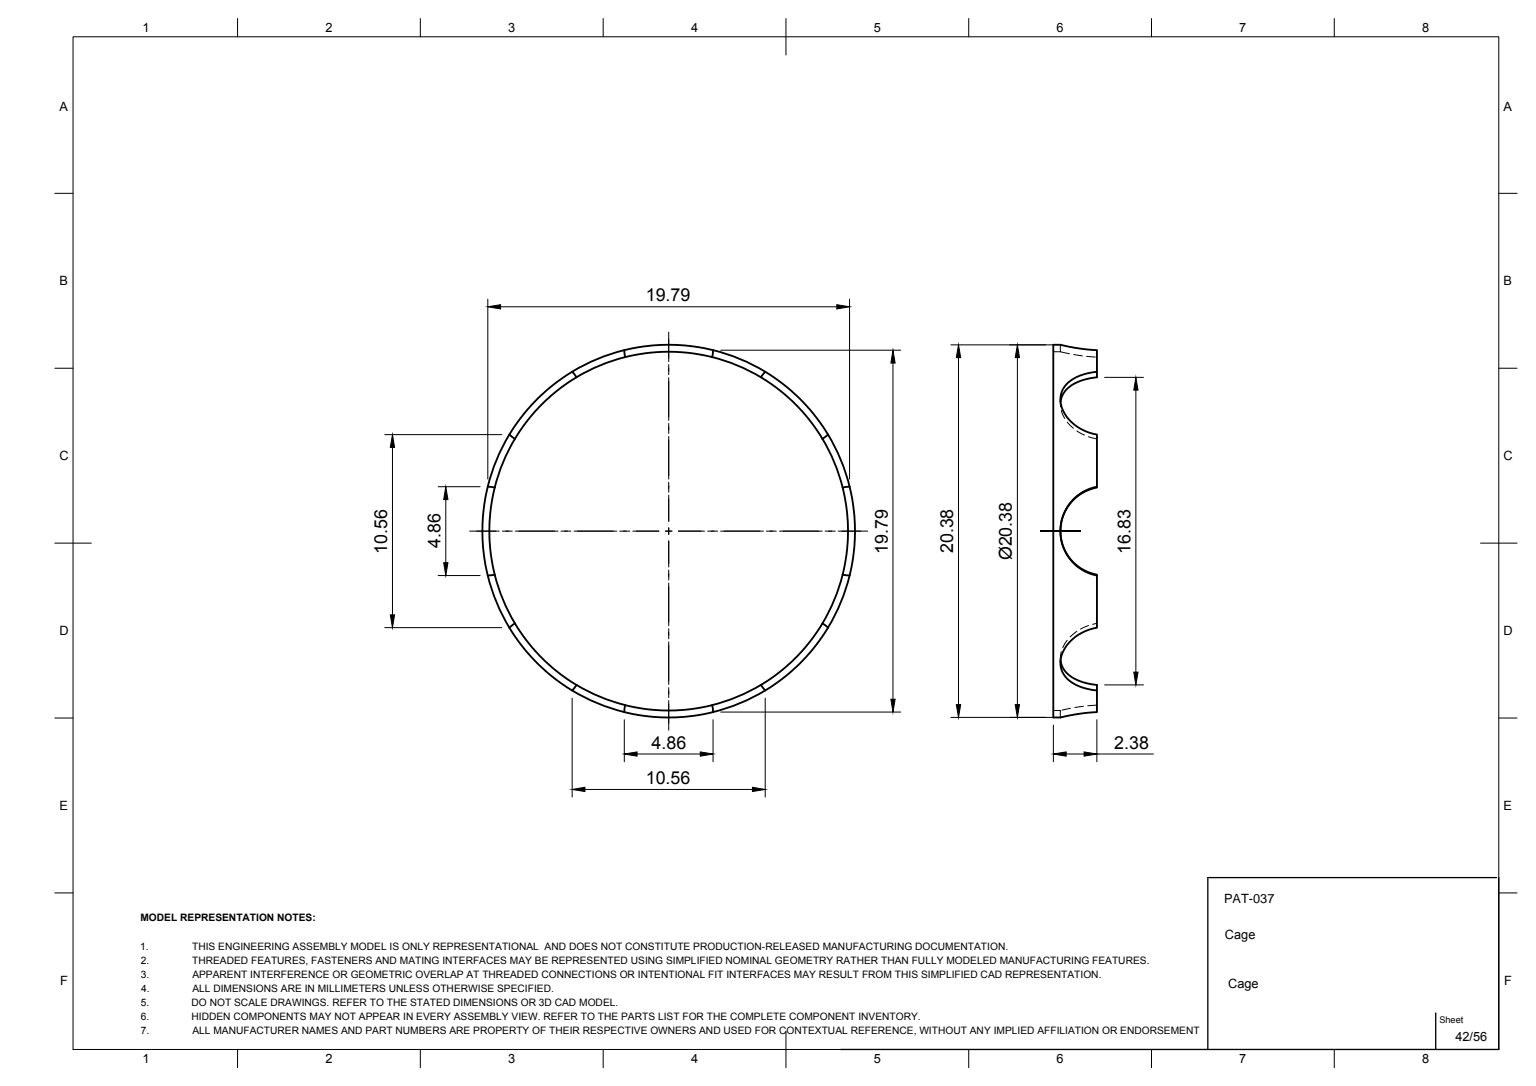
ISO-10303-21;
HEADER;
/* Generated by software containing ST-Developer
 * from STEP Tools, Inc. (www.steptools.com) 
 */

FILE_DESCRIPTION(
/* description */ ('Flywheel Crank-Slider'),
/* implementation_level */ '2;1');

FILE_NAME(
/* name */ 'Cage.step',
/* time_stamp */ '2026-10-28T03:23:13-07:00',
/* author */ (''),
/* organization */ (''),
/* preprocessor_version */ 'ST-DEVELOPER v20.2',
/* originating_system */ 'Autodesk Translation Framework v15.17.0.0',
/* authorisation */ '');

FILE_SCHEMA (('AUTOMOTIVE_DESIGN { 1 0 10303 214 3 1 1 }'));
ENDSEC;

DATA;
#10=MECHANICAL_DESIGN_GEOMETRIC_PRESENTATION_REPRESENTATION('',(#716),#17322);
#493=B_SPLINE_CURVE_WITH_KNOTS('',3,(#16156,#16157,#16158,#16159,#16160,
#16161,#16162,#16163,#16164,#16165,#16166,#16167,#16168,#16169,#16170,#16171,
#16172,#16173,#16174,#16175,#16176,#16177),.UNSPECIFIED.,.F.,.F.,(4,2,2,
2,2,2,2,2,2,2,4),(0.0473477652366656,0.126350602536658,0.189525903804987,
0.252701205073317,0.313298422430275,0.373895639787233,0.434492857144191,
0.495090074501149,0.558265375769478,0.621440677037807,0.7004435143378),
 .UNSPECIFIED.);
#494=B_SPLINE_CURVE_WITH_KNOTS('',3,(#16181,#16182,#16183,#16184,#16185,
#16186,#16187,#16188,#16189,#16190,#16191,#16192,#16193,#16194,#16195,#16196,
#16197,#16198,#16199,#16200,#16201,#16202),.UNSPECIFIED.,.F.,.F.,(4,2,2,
2,2,2,2,2,2,2,4),(0.0464897534940957,0.0852567806515119,0.170513561303024,
0.246687263103517,0.308657850341199,0.370628437578881,0.432599024816563,
0.494569612054245,0.570743313854739,0.656000094506251,0.694767121663666),
 .UNSPECIFIED.);
#495=B_SPLINE_CURVE_WITH_KNOTS('',3,(#16208,#16209,#16210,#16211,#16212,
#16213,#16214,#16215,#16216,#16217,#16218,#16219,#16220,#16221,#16222,#16223,
#16224,#16225,#16226,#16227,#16228,#16229),.UNSPECIFIED.,.F.,.F.,(4,2,2,
2,2,2,2,2,2,2,4),(0.0464897534940957,0.0852567806515118,0.170513561303024,
0.246687263103517,0.308657850341199,0.370628437578881,0.432599024816563,
0.494569612054245,0.570743313854738,0.65600009450625,0.694767121663666),
 .UNSPECIFIED.);
#496=B_SPLINE_CURVE_WITH_KNOTS('',3,(#16233,#16234,#16235,#16236,#16237,
#16238,#16239,#16240,#16241,#16242,#16243,#16244,#16245,#16246,#16247,#16248,
#16249,#16250,#16251,#16252,#16253,#16254),.UNSPECIFIED.,.F.,.F.,(4,2,2,
2,2,2,2,2,2,2,4),(0.0464897534940957,0.0852567806515119,0.170513561303024,
0.246687263103517,0.308657850341199,0.370628437578881,0.432599024816563,
0.494569612054245,0.570743313854739,0.656000094506251,0.694767121663666),
 .UNSPECIFIED.);
#497=B_SPLINE_CURVE_WITH_KNOTS('',3,(#16258,#16259,#16260,#16261,#16262,
#16263,#16264,#16265,#16266,#16267,#16268,#16269),.UNSPECIFIED.,.F.,.F.,
(4,2,2,2,2,4),(0.0464897534940957,0.0852567806515119,0.170513561303024,
0.246687263103517,0.308657850341199,0.370628437578881),.UNSPECIFIED.);
#498=B_SPLINE_CURVE_WITH_KNOTS('',3,(#16274,#16275,#16276,#16277,#16278,
#16279,#16280,#16281,#16282,#16283,#16284,#16285),.UNSPECIFIED.,.F.,.F.,
(4,2,2,2,2,4),(0.370628437578881,0.432599024816563,0.494569612054245,0.570743313854738,
0.65600009450625,0.694767121663666),.UNSPECIFIED.);
#499=B_SPLINE_CURVE_WITH_KNOTS('',3,(#16289,#16290,#16291,#16292,#16293,
#16294,#16295,#16296,#16297,#16298,#16299,#16300,#16301,#16302,#16303,#16304,
#16305,#16306,#16307,#16308,#16309,#16310),.UNSPECIFIED.,.F.,.F.,(4,2,2,
2,2,2,2,2,2,2,4),(0.0464897534940957,0.0852567806515121,0.170513561303024,
0.246687263103518,0.308657850341199,0.370628437578881,0.432599024816563,
0.494569612054245,0.570743313854738,0.65600009450625,0.694767121663666),
 .UNSPECIFIED.);
#500=B_SPLINE_CURVE_WITH_KNOTS('',3,(#16314,#16315,#16316,#16317,#16318,
#16319,#16320,#16321,#16322,#16323,#16324,#16325,#16326,#16327,#16328,#16329,
#16330,#16331,#16332,#16333,#16334,#16335),.UNSPECIFIED.,.F.,.F.,(4,2,2,
2,2,2,2,2,2,2,4),(0.0464897534940957,0.0852567806515119,0.170513561303024,
0.246687263103517,0.308657850341199,0.370628437578881,0.432599024816563,
0.494569612054245,0.570743313854738,0.65600009450625,0.694767121663667),
 .UNSPECIFIED.);
#501=B_SPLINE_CURVE_WITH_KNOTS('',3,(#16339,#16340,#16341,#16342,#16343,
#16344,#16345,#16346,#16347,#16348,#16349,#16350,#16351,#16352,#16353,#16354,
#16355,#16356,#16357,#16358,#16359,#16360),.UNSPECIFIED.,.F.,.F.,(4,2,2,
2,2,2,2,2,2,2,4),(0.0464897534940957,0.0852567806515119,0.170513561303024,
0.246687263103517,0.308657850341199,0.370628437578881,0.432599024816563,
0.494569612054245,0.570743313854738,0.65600009450625,0.694767121663666),
 .UNSPECIFIED.);
#502=B_SPLINE_CURVE_WITH_KNOTS('',3,(#16364,#16365,#16366,#16367,#16368,
#16369,#16370,#16371,#16372,#16373,#16374,#16375,#16376,#16377,#16378,#16379,
#16380,#16381,#16382,#16383,#16384,#16385),.UNSPECIFIED.,.F.,.F.,(4,2,2,
2,2,2,2,2,2,2,4),(0.0464897534940957,0.0852567806515119,0.170513561303024,
0.246687263103517,0.308657850341199,0.370628437578881,0.432599024816563,
0.494569612054245,0.570743313854739,0.656000094506251,0.694767121663667),
 .UNSPECIFIED.);
#503=B_SPLINE_CURVE_WITH_KNOTS('',3,(#16393,#16394,#16395,#16396,#16397,
#16398,#16399,#16400,#16401,#16402,#16403,#16404,#16405,#16406,#16407,#16408,
#16409,#16410,#16411,#16412,#16413,#16414),.UNSPECIFIED.,.F.,.F.,(4,2,2,
2,2,2,2,2,2,2,4),(0.0473477652366656,0.126350602536658,0.189525903804987,
0.252701205073316,0.313298422430274,0.373895639787232,0.434492857144191,
0.495090074501149,0.558265375769478,0.621440677037807,0.7004435143378),
 .UNSPECIFIED.);
#504=B_SPLINE_CURVE_WITH_KNOTS('',3,(#16422,#16423,#16424,#16425,#16426,
#16427,#16428,#16429,#16430,#16431,#16432,#16433,#16434,#16435,#16436,#16437,
#16438,#16439,#16440,#16441,#16442,#16443),.UNSPECIFIED.,.F.,.F.,(4,2,2,
2,2,2,2,2,2,2,4),(0.0473477652366656,0.126350602536658,0.189525903804987,
0.252701205073317,0.313298422430275,0.373895639787233,0.434492857144191,
0.495090074501149,0.558265375769478,0.621440677037807,0.7004435143378),
 .UNSPECIFIED.);
#505=B_SPLINE_CURVE_WITH_KNOTS('',3,(#16452,#16453,#16454,#16455,#16456,
#16457,#16458,#16459,#16460,#16461,#16462,#16463),.UNSPECIFIED.,.F.,.F.,
(4,2,2,2,2,4),(0.0473477652366656,0.126350602536658,0.189525903804987,0.252701205073316,
0.313298422430275,0.373895639787233),.UNSPECIFIED.);
#506=B_SPLINE_CURVE_WITH_KNOTS('',3,(#16465,#16466,#16467,#16468,#16469,
#16470,#16471,#16472,#16473,#16474,#16475,#16476),.UNSPECIFIED.,.F.,.F.,
(4,2,2,2,2,4),(0.373895639787233,0.434492857144191,0.495090074501149,0.558265375769478,
0.621440677037807,0.7004435143378),.UNSPECIFIED.);
#507=B_SPLINE_CURVE_WITH_KNOTS('',3,(#16483,#16484,#16485,#16486,#16487,
#16488,#16489,#16490,#16491,#16492,#16493,#16494,#16495,#16496,#16497,#16498,
#16499,#16500,#16501,#16502,#16503,#16504),.UNSPECIFIED.,.F.,.F.,(4,2,2,
2,2,2,2,2,2,2,4),(0.0473477652366656,0.126350602536658,0.189525903804987,
0.252701205073316,0.313298422430275,0.373895639787233,0.434492857144191,
0.495090074501149,0.558265375769478,0.621440677037807,0.7004435143378),
 .UNSPECIFIED.);
#508=B_SPLINE_CURVE_WITH_KNOTS('',3,(#16512,#16513,#16514,#16515,#16516,
#16517,#16518,#16519,#16520,#16521,#16522,#16523,#16524,#16525,#16526,#16527,
#16528,#16529,#16530,#16531,#16532,#16533),.UNSPECIFIED.,.F.,.F.,(4,2,2,
2,2,2,2,2,2,2,4),(0.0473477652366656,0.126350602536658,0.189525903804987,
0.252701205073317,0.313298422430275,0.373895639787233,0.434492857144191,
0.495090074501149,0.558265375769478,0.621440677037807,0.7004435143378),
 .UNSPECIFIED.);
#509=B_SPLINE_CURVE_WITH_KNOTS('',3,(#16541,#16542,#16543,#16544,#16545,
#16546,#16547,#16548,#16549,#16550,#16551,#16552,#16553,#16554,#16555,#16556,
#16557,#16558,#16559,#16560,#16561,#16562),.UNSPECIFIED.,.F.,.F.,(4,2,2,
2,2,2,2,2,2,2,4),(0.0473477652366656,0.126350602536658,0.189525903804987,
0.252701205073316,0.313298422430275,0.373895639787233,0.434492857144191,
0.495090074501149,0.558265375769478,0.621440677037807,0.7004435143378),
 .UNSPECIFIED.);
#510=B_SPLINE_CURVE_WITH_KNOTS('',3,(#16571,#16572,#16573,#16574,#16575,
#16576,#16577,#16578,#16579,#16580,#16581,#16582,#16583,#16584,#16585,#16586,
#16587,#16588,#16589,#16590,#16591,#16592),.UNSPECIFIED.,.F.,.F.,(4,2,2,
2,2,2,2,2,2,2,4),(0.0473477652366656,0.126350602536658,0.189525903804987,
0.252701205073317,0.313298422430275,0.373895639787233,0.434492857144191,
0.495090074501149,0.558265375769478,0.621440677037807,0.7004435143378),
 .UNSPECIFIED.);
#521=SPHERICAL_SURFACE('',#10452,0.247676);
#522=SPHERICAL_SURFACE('',#10468,0.247676);
#523=SPHERICAL_SURFACE('',#10473,0.247676);
#524=SPHERICAL_SURFACE('',#10478,0.247676);
#525=SPHERICAL_SURFACE('',#10483,0.247676);
#526=SPHERICAL_SURFACE('',#10488,0.247676);
#527=SPHERICAL_SURFACE('',#10493,0.247676);
#528=SPHERICAL_SURFACE('',#10501,0.247676);
#604=SHAPE_REPRESENTATION_RELATIONSHIP('SRR','None',#17604,#656);
#656=ADVANCED_BREP_SHAPE_REPRESENTATION('',(#773),#17308);
#716=STYLED_ITEM('',(#17931),#773);
#773=MANIFOLD_SOLID_BREP('Continuous crown cage',#9098);
#947=FACE_BOUND('',#2441,.T.);
#1246=PLANE('',#10465);
#1247=PLANE('',#10470);
#1248=PLANE('',#10475);
#1249=PLANE('',#10480);
#1250=PLANE('',#10485);
#1251=PLANE('',#10490);
#1252=PLANE('',#10499);
#1253=PLANE('',#10503);
#1254=PLANE('',#10504);
#1726=FACE_OUTER_BOUND('',#2423,.T.);
#1727=FACE_OUTER_BOUND('',#2424,.T.);
#1728=FACE_OUTER_BOUND('',#2425,.T.);
#1729=FACE_OUTER_BOUND('',#2426,.T.);
#1730=FACE_OUTER_BOUND('',#2427,.T.);
#1731=FACE_OUTER_BOUND('',#2428,.T.);
#1732=FACE_OUTER_BOUND('',#2429,.T.);
#1733=FACE_OUTER_BOUND('',#2430,.T.);
#1734=FACE_OUTER_BOUND('',#2431,.T.);
#1735=FACE_OUTER_BOUND('',#2432,.T.);
#1736=FACE_OUTER_BOUND('',#2433,.T.);
#1737=FACE_OUTER_BOUND('',#2434,.T.);
#1738=FACE_OUTER_BOUND('',#2435,.T.);
#1739=FACE_OUTER_BOUND('',#2436,.T.);
#1740=FACE_OUTER_BOUND('',#2437,.T.);
#1741=FACE_OUTER_BOUND('',#2438,.T.);
#1742=FACE_OUTER_BOUND('',#2439,.T.);
#1743=FACE_OUTER_BOUND('',#2440,.T.);
#1744=FACE_OUTER_BOUND('',#2442,.T.);
#2423=EDGE_LOOP('',(#7778,#7779,#7780,#7781));
#2424=EDGE_LOOP('',(#7782,#7783,#7784,#7785,#7786,#7787,#7788,#7789,#7790,
#7791,#7792,#7793,#7794,#7795,#7796,#7797,#7798,#7799,#7800,#7801));
#2425=EDGE_LOOP('',(#7802,#7803,#7804,#7805));
#2426=EDGE_LOOP('',(#7806,#7807,#7808,#7809));
#2427=EDGE_LOOP('',(#7810,#7811,#7812,#7813));
#2428=EDGE_LOOP('',(#7814,#7815,#7816,#7817));
#2429=EDGE_LOOP('',(#7818,#7819,#7820,#7821));
#2430=EDGE_LOOP('',(#7822,#7823,#7824,#7825,#7826,#7827));
#2431=EDGE_LOOP('',(#7828,#7829,#7830,#7831));
#2432=EDGE_LOOP('',(#7832,#7833,#7834,#7835));
#2433=EDGE_LOOP('',(#7836,#7837,#7838,#7839));
#2434=EDGE_LOOP('',(#7840,#7841,#7842,#7843));
#2435=EDGE_LOOP('',(#7844,#7845,#7846,#7847));
#2436=EDGE_LOOP('',(#7848,#7849,#7850,#7851));
#2437=EDGE_LOOP('',(#7852,#7853,#7854,#7855,#7856,#7857,#7858,#7859,#7860,
#7861,#7862,#7863,#7864,#7865,#7866,#7867,#7868,#7869,#7870,#7871));
#2438=EDGE_LOOP('',(#7872,#7873,#7874,#7875));
#2439=EDGE_LOOP('',(#7876,#7877,#7878,#7879));
#2440=EDGE_LOOP('',(#7880));
#2441=EDGE_LOOP('',(#7881));
#2442=EDGE_LOOP('',(#7882,#7883,#7884,#7885));
#3096=LINE('',#16271,#3707);
#3097=LINE('',#16567,#3708);
#3707=VECTOR('',#12858,1.019052);
#3708=VECTOR('',#12935,0.980948);
#4150=CIRCLE('',#10453,0.243053047864041);
#4151=CIRCLE('',#10454,0.243053047864041);
#4152=CIRCLE('',#10456,1.019052);
#4153=CIRCLE('',#10457,1.019052);
#4154=CIRCLE('',#10458,1.019052);
#4155=CIRCLE('',#10459,1.019052);
#4156=CIRCLE('',#10460,1.019052);
#4157=CIRCLE('',#10461,1.019052);
#4158=CIRCLE('',#10462,1.019052);
#4159=CIRCLE('',#10463,1.019052);
#4160=CIRCLE('',#10464,1.019052);
#4161=CIRCLE('',#10466,0.980948);
#4162=CIRCLE('',#10467,0.243053047864041);
#4163=CIRCLE('',#10469,0.243053047864041);
#4164=CIRCLE('',#10471,0.980948);
#4165=CIRCLE('',#10472,0.243053047864041);
#4166=CIRCLE('',#10474,0.243053047864041);
#4167=CIRCLE('',#10476,0.980948);
#4168=CIRCLE('',#10477,0.243053047864041);
#4169=CIRCLE('',#10479,0.243053047864041);
#4170=CIRCLE('',#10481,0.980948);
#4171=CIRCLE('',#10482,0.243053047864041);
#4172=CIRCLE('',#10484,0.243053047864041);
#4173=CIRCLE('',#10486,0.980948);
#4174=CIRCLE('',#10487,0.243053047864041);
#4175=CIRCLE('',#10489,0.243053047864041);
#4176=CIRCLE('',#10491,0.980948);
#4177=CIRCLE('',#10492,0.243053047864041);
#4178=CIRCLE('',#10494,0.243053047864041);
#4179=CIRCLE('',#10496,0.980948);
#4180=CIRCLE('',#10497,0.980948);
#4181=CIRCLE('',#10498,0.980948);
#4182=CIRCLE('',#10500,0.243053047864041);
#4183=CIRCLE('',#10502,0.243053047864041);
#4835=VERTEX_POINT('',#16154);
#4836=VERTEX_POINT('',#16155);
#4837=VERTEX_POINT('',#16178);
#4838=VERTEX_POINT('',#16180);
#4839=VERTEX_POINT('',#16205);
#4840=VERTEX_POINT('',#16207);
#4841=VERTEX_POINT('',#16230);
#4842=VERTEX_POINT('',#16232);
#4843=VERTEX_POINT('',#16255);
#4844=VERTEX_POINT('',#16257);
#4845=VERTEX_POINT('',#16270);
#4846=VERTEX_POINT('',#16273);
#4847=VERTEX_POINT('',#16286);
#4848=VERTEX_POINT('',#16288);
#4849=VERTEX_POINT('',#16311);
#4850=VERTEX_POINT('',#16313);
#4851=VERTEX_POINT('',#16336);
#4852=VERTEX_POINT('',#16338);
#4853=VERTEX_POINT('',#16361);
#4854=VERTEX_POINT('',#16363);
#4855=VERTEX_POINT('',#16388);
#4856=VERTEX_POINT('',#16392);
#4857=VERTEX_POINT('',#16417);
#4858=VERTEX_POINT('',#16421);
#4859=VERTEX_POINT('',#16446);
#4860=VERTEX_POINT('',#16450);
#4861=VERTEX_POINT('',#16451);
#4862=VERTEX_POINT('',#16478);
#4863=VERTEX_POINT('',#16482);
#4864=VERTEX_POINT('',#16507);
#4865=VERTEX_POINT('',#16511);
#4866=VERTEX_POINT('',#16536);
#4867=VERTEX_POINT('',#16540);
#4868=VERTEX_POINT('',#16565);
#4869=VERTEX_POINT('',#16568);
#4870=VERTEX_POINT('',#16570);
#5846=EDGE_CURVE('',#4835,#4836,#493,.T.);
#5847=EDGE_CURVE('',#4837,#4835,#4150,.T.);
#5848=EDGE_CURVE('',#4838,#4837,#494,.T.);
#5849=EDGE_CURVE('',#4836,#4838,#4151,.T.);
#5850=EDGE_CURVE('',#4839,#4837,#4152,.T.);
#5851=EDGE_CURVE('',#4839,#4840,#495,.T.);
#5852=EDGE_CURVE('',#4841,#4840,#4153,.T.);
#5853=EDGE_CURVE('',#4841,#4842,#496,.T.);
#5854=EDGE_CURVE('',#4843,#4842,#4154,.T.);
#5855=EDGE_CURVE('',#4843,#4844,#497,.T.);
#5856=EDGE_CURVE('',#4844,#4845,#3096,.T.);
#5857=EDGE_CURVE('',#4845,#4845,#4155,.T.);
#5858=EDGE_CURVE('',#4844,#4846,#498,.T.);
#5859=EDGE_CURVE('',#4847,#4846,#4156,.T.);
#5860=EDGE_CURVE('',#4847,#4848,#499,.T.);
#5861=EDGE_CURVE('',#4849,#4848,#4157,.T.);
#5862=EDGE_CURVE('',#4849,#4850,#500,.T.);
#5863=EDGE_CURVE('',#4851,#4850,#4158,.T.);
#5864=EDGE_CURVE('',#4851,#4852,#501,.T.);
#5865=EDGE_CURVE('',#4853,#4852,#4159,.T.);
#5866=EDGE_CURVE('',#4853,#4854,#502,.T.);
#5867=EDGE_CURVE('',#4838,#4854,#4160,.T.);
#5868=EDGE_CURVE('',#4835,#4855,#4161,.T.);
#5869=EDGE_CURVE('',#4855,#4839,#4162,.T.);
#5870=EDGE_CURVE('',#4856,#4855,#503,.T.);
#5871=EDGE_CURVE('',#4840,#4856,#4163,.T.);
#5872=EDGE_CURVE('',#4856,#4857,#4164,.T.);
#5873=EDGE_CURVE('',#4857,#4841,#4165,.T.);
#5874=EDGE_CURVE('',#4858,#4857,#504,.T.);
#5875=EDGE_CURVE('',#4842,#4858,#4166,.T.);
#5876=EDGE_CURVE('',#4858,#4859,#4167,.T.);
#5877=EDGE_CURVE('',#4859,#4843,#4168,.T.);
#5878=EDGE_CURVE('',#4860,#4861,#505,.T.);
#5879=EDGE_CURVE('',#4846,#4860,#4169,.T.);
#5880=EDGE_CURVE('',#4861,#4859,#506,.T.);
#5881=EDGE_CURVE('',#4860,#4862,#4170,.T.);
#5882=EDGE_CURVE('',#4862,#4847,#4171,.T.);
#5883=EDGE_CURVE('',#4863,#4862,#507,.T.);
#5884=EDGE_CURVE('',#4848,#4863,#4172,.T.);
#5885=EDGE_CURVE('',#4863,#4864,#4173,.T.);
#5886=EDGE_CURVE('',#4864,#4849,#4174,.T.);
#5887=EDGE_CURVE('',#4865,#4864,#508,.T.);
#5888=EDGE_CURVE('',#4850,#4865,#4175,.T.);
#5889=EDGE_CURVE('',#4865,#4866,#4176,.T.);
#5890=EDGE_CURVE('',#4866,#4851,#4177,.T.);
#5891=EDGE_CURVE('',#4867,#4866,#509,.T.);
#5892=EDGE_CURVE('',#4852,#4867,#4178,.T.);
#5893=EDGE_CURVE('',#4868,#4868,#4179,.T.);
#5894=EDGE_CURVE('',#4868,#4861,#3097,.T.);
#5895=EDGE_CURVE('',#4869,#4836,#4180,.T.);
#5896=EDGE_CURVE('',#4869,#4870,#510,.T.);
#5897=EDGE_CURVE('',#4867,#4870,#4181,.T.);
#5898=EDGE_CURVE('',#4854,#4869,#4182,.T.);
#5899=EDGE_CURVE('',#4870,#4853,#4183,.T.);
#7778=ORIENTED_EDGE('',*,*,#5846,.F.);
#7779=ORIENTED_EDGE('',*,*,#5847,.F.);
#7780=ORIENTED_EDGE('',*,*,#5848,.F.);
#7781=ORIENTED_EDGE('',*,*,#5849,.F.);
#7782=ORIENTED_EDGE('',*,*,#5848,.T.);
#7783=ORIENTED_EDGE('',*,*,#5850,.F.);
#7784=ORIENTED_EDGE('',*,*,#5851,.T.);
#7785=ORIENTED_EDGE('',*,*,#5852,.F.);
#7786=ORIENTED_EDGE('',*,*,#5853,.T.);
#7787=ORIENTED_EDGE('',*,*,#5854,.F.);
#7788=ORIENTED_EDGE('',*,*,#5855,.T.);
#7789=ORIENTED_EDGE('',*,*,#5856,.T.);
#7790=ORIENTED_EDGE('',*,*,#5857,.F.);
#7791=ORIENTED_EDGE('',*,*,#5856,.F.);
#7792=ORIENTED_EDGE('',*,*,#5858,.T.);
#7793=ORIENTED_EDGE('',*,*,#5859,.F.);
#7794=ORIENTED_EDGE('',*,*,#5860,.T.);
#7795=ORIENTED_EDGE('',*,*,#5861,.F.);
#7796=ORIENTED_EDGE('',*,*,#5862,.T.);
#7797=ORIENTED_EDGE('',*,*,#5863,.F.);
#7798=ORIENTED_EDGE('',*,*,#5864,.T.);
#7799=ORIENTED_EDGE('',*,*,#5865,.F.);
#7800=ORIENTED_EDGE('',*,*,#5866,.T.);
#7801=ORIENTED_EDGE('',*,*,#5867,.F.);
#7802=ORIENTED_EDGE('',*,*,#5847,.T.);
#7803=ORIENTED_EDGE('',*,*,#5868,.T.);
#7804=ORIENTED_EDGE('',*,*,#5869,.T.);
#7805=ORIENTED_EDGE('',*,*,#5850,.T.);
#7806=ORIENTED_EDGE('',*,*,#5870,.F.);
#7807=ORIENTED_EDGE('',*,*,#5871,.F.);
#7808=ORIENTED_EDGE('',*,*,#5851,.F.);
#7809=ORIENTED_EDGE('',*,*,#5869,.F.);
#7810=ORIENTED_EDGE('',*,*,#5871,.T.);
#7811=ORIENTED_EDGE('',*,*,#5872,.T.);
#7812=ORIENTED_EDGE('',*,*,#5873,.T.);
#7813=ORIENTED_EDGE('',*,*,#5852,.T.);
#7814=ORIENTED_EDGE('',*,*,#5874,.F.);
#7815=ORIENTED_EDGE('',*,*,#5875,.F.);
#7816=ORIENTED_EDGE('',*,*,#5853,.F.);
#7817=ORIENTED_EDGE('',*,*,#5873,.F.);
#7818=ORIENTED_EDGE('',*,*,#5875,.T.);
#7819=ORIENTED_EDGE('',*,*,#5876,.T.);
#7820=ORIENTED_EDGE('',*,*,#5877,.T.);
#7821=ORIENTED_EDGE('',*,*,#5854,.T.);
#7822=ORIENTED_EDGE('',*,*,#5878,.F.);
#7823=ORIENTED_EDGE('',*,*,#5879,.F.);
#7824=ORIENTED_EDGE('',*,*,#5858,.F.);
#7825=ORIENTED_EDGE('',*,*,#5855,.F.);
#7826=ORIENTED_EDGE('',*,*,#5877,.F.);
#7827=ORIENTED_EDGE('',*,*,#5880,.F.);
#7828=ORIENTED_EDGE('',*,*,#5879,.T.);
#7829=ORIENTED_EDGE('',*,*,#5881,.T.);
#7830=ORIENTED_EDGE('',*,*,#5882,.T.);
#7831=ORIENTED_EDGE('',*,*,#5859,.T.);
#7832=ORIENTED_EDGE('',*,*,#5883,.F.);
#7833=ORIENTED_EDGE('',*,*,#5884,.F.);
#7834=ORIENTED_EDGE('',*,*,#5860,.F.);
#7835=ORIENTED_EDGE('',*,*,#5882,.F.);
#7836=ORIENTED_EDGE('',*,*,#5884,.T.);
#7837=ORIENTED_EDGE('',*,*,#5885,.T.);
#7838=ORIENTED_EDGE('',*,*,#5886,.T.);
#7839=ORIENTED_EDGE('',*,*,#5861,.T.);
#7840=ORIENTED_EDGE('',*,*,#5887,.F.);
#7841=ORIENTED_EDGE('',*,*,#5888,.F.);
#7842=ORIENTED_EDGE('',*,*,#5862,.F.);
#7843=ORIENTED_EDGE('',*,*,#5886,.F.);
#7844=ORIENTED_EDGE('',*,*,#5888,.T.);
#7845=ORIENTED_EDGE('',*,*,#5889,.T.);
#7846=ORIENTED_EDGE('',*,*,#5890,.T.);
#7847=ORIENTED_EDGE('',*,*,#5863,.T.);
#7848=ORIENTED_EDGE('',*,*,#5864,.F.);
#7849=ORIENTED_EDGE('',*,*,#5890,.F.);
#7850=ORIENTED_EDGE('',*,*,#5891,.F.);
#7851=ORIENTED_EDGE('',*,*,#5892,.F.);
#7852=ORIENTED_EDGE('',*,*,#5893,.F.);
#7853=ORIENTED_EDGE('',*,*,#5894,.T.);
#7854=ORIENTED_EDGE('',*,*,#5880,.T.);
#7855=ORIENTED_EDGE('',*,*,#5876,.F.);
#7856=ORIENTED_EDGE('',*,*,#5874,.T.);
#7857=ORIENTED_EDGE('',*,*,#5872,.F.);
#7858=ORIENTED_EDGE('',*,*,#5870,.T.);
#7859=ORIENTED_EDGE('',*,*,#5868,.F.);
#7860=ORIENTED_EDGE('',*,*,#5846,.T.);
#7861=ORIENTED_EDGE('',*,*,#5895,.F.);
#7862=ORIENTED_EDGE('',*,*,#5896,.T.);
#7863=ORIENTED_EDGE('',*,*,#5897,.F.);
#7864=ORIENTED_EDGE('',*,*,#5891,.T.);
#7865=ORIENTED_EDGE('',*,*,#5889,.F.);
#7866=ORIENTED_EDGE('',*,*,#5887,.T.);
#7867=ORIENTED_EDGE('',*,*,#5885,.F.);
#7868=ORIENTED_EDGE('',*,*,#5883,.T.);
#7869=ORIENTED_EDGE('',*,*,#5881,.F.);
#7870=ORIENTED_EDGE('',*,*,#5878,.T.);
#7871=ORIENTED_EDGE('',*,*,#5894,.F.);
#7872=ORIENTED_EDGE('',*,*,#5849,.T.);
#7873=ORIENTED_EDGE('',*,*,#5867,.T.);
#7874=ORIENTED_EDGE('',*,*,#5898,.T.);
#7875=ORIENTED_EDGE('',*,*,#5895,.T.);
#7876=ORIENTED_EDGE('',*,*,#5866,.F.);
#7877=ORIENTED_EDGE('',*,*,#5899,.F.);
#7878=ORIENTED_EDGE('',*,*,#5896,.F.);
#7879=ORIENTED_EDGE('',*,*,#5898,.F.);
#7880=ORIENTED_EDGE('',*,*,#5857,.T.);
#7881=ORIENTED_EDGE('',*,*,#5893,.T.);
#7882=ORIENTED_EDGE('',*,*,#5892,.T.);
#7883=ORIENTED_EDGE('',*,*,#5897,.T.);
#7884=ORIENTED_EDGE('',*,*,#5899,.T.);
#7885=ORIENTED_EDGE('',*,*,#5865,.T.);
#8467=CYLINDRICAL_SURFACE('',#10455,1.019052);
#8468=CYLINDRICAL_SURFACE('',#10495,0.980948);
#8917=ADVANCED_FACE('',(#1726),#521,.F.);
#8918=ADVANCED_FACE('',(#1727),#8467,.T.);
#8919=ADVANCED_FACE('',(#1728),#1246,.T.);
#8920=ADVANCED_FACE('',(#1729),#522,.F.);
#8921=ADVANCED_FACE('',(#1730),#1247,.T.);
#8922=ADVANCED_FACE('',(#1731),#523,.F.);
#8923=ADVANCED_FACE('',(#1732),#1248,.T.);
#8924=ADVANCED_FACE('',(#1733),#524,.F.);
#8925=ADVANCED_FACE('',(#1734),#1249,.T.);
#8926=ADVANCED_FACE('',(#1735),#525,.F.);
#8927=ADVANCED_FACE('',(#1736),#1250,.T.);
#8928=ADVANCED_FACE('',(#1737),#526,.F.);
#8929=ADVANCED_FACE('',(#1738),#1251,.T.);
#8930=ADVANCED_FACE('',(#1739),#527,.F.);
#8931=ADVANCED_FACE('',(#1740),#8468,.F.);
#8932=ADVANCED_FACE('',(#1741),#1252,.T.);
#8933=ADVANCED_FACE('',(#1742),#528,.F.);
#8934=ADVANCED_FACE('',(#1743,#947),#1253,.T.);
#8935=ADVANCED_FACE('',(#1744),#1254,.T.);
#9098=CLOSED_SHELL('',(#8917,#8918,#8919,#8920,#8921,#8922,#8923,#8924,
#8925,#8926,#8927,#8928,#8929,#8930,#8931,#8932,#8933,#8934,#8935));
#10451=AXIS2_PLACEMENT_3D('',#16152,#12842,#12843);
#10452=AXIS2_PLACEMENT_3D('',#16153,#12844,#12845);
#10453=AXIS2_PLACEMENT_3D('',#16179,#12846,#12847);
#10454=AXIS2_PLACEMENT_3D('',#16203,#12848,#12849);
#10455=AXIS2_PLACEMENT_3D('',#16204,#12850,#12851);
#10456=AXIS2_PLACEMENT_3D('',#16206,#12852,#12853);
#10457=AXIS2_PLACEMENT_3D('',#16231,#12854,#12855);
#10458=AXIS2_PLACEMENT_3D('',#16256,#12856,#12857);
#10459=AXIS2_PLACEMENT_3D('',#16272,#12859,#12860);
#10460=AXIS2_PLACEMENT_3D('',#16287,#12861,#12862);
#10461=AXIS2_PLACEMENT_3D('',#16312,#12863,#12864);
#10462=AXIS2_PLACEMENT_3D('',#16337,#12865,#12866);
#10463=AXIS2_PLACEMENT_3D('',#16362,#12867,#12868);
#10464=AXIS2_PLACEMENT_3D('',#16386,#12869,#12870);
#10465=AXIS2_PLACEMENT_3D('',#16387,#12871,#12872);
#10466=AXIS2_PLACEMENT_3D('',#16389,#12873,#12874);
#10467=AXIS2_PLACEMENT_3D('',#16390,#12875,#12876);
#10468=AXIS2_PLACEMENT_3D('',#16391,#12877,#12878);
#10469=AXIS2_PLACEMENT_3D('',#16415,#12879,#12880);
#10470=AXIS2_PLACEMENT_3D('',#16416,#12881,#12882);
#10471=AXIS2_PLACEMENT_3D('',#16418,#12883,#12884);
#10472=AXIS2_PLACEMENT_3D('',#16419,#12885,#12886);
#10473=AXIS2_PLACEMENT_3D('',#16420,#12887,#12888);
#10474=AXIS2_PLACEMENT_3D('',#16444,#12889,#12890);
#10475=AXIS2_PLACEMENT_3D('',#16445,#12891,#12892);
#10476=AXIS2_PLACEMENT_3D('',#16447,#12893,#12894);
#10477=AXIS2_PLACEMENT_3D('',#16448,#12895,#12896);
#10478=AXIS2_PLACEMENT_3D('',#16449,#12897,#12898);
#10479=AXIS2_PLACEMENT_3D('',#16464,#12899,#12900);
#10480=AXIS2_PLACEMENT_3D('',#16477,#12901,#12902);
#10481=AXIS2_PLACEMENT_3D('',#16479,#12903,#12904);
#10482=AXIS2_PLACEMENT_3D('',#16480,#12905,#12906);
#10483=AXIS2_PLACEMENT_3D('',#16481,#12907,#12908);
#10484=AXIS2_PLACEMENT_3D('',#16505,#12909,#12910);
#10485=AXIS2_PLACEMENT_3D('',#16506,#12911,#12912);
#10486=AXIS2_PLACEMENT_3D('',#16508,#12913,#12914);
#10487=AXIS2_PLACEMENT_3D('',#16509,#12915,#12916);
#10488=AXIS2_PLACEMENT_3D('',#16510,#12917,#12918);
#10489=AXIS2_PLACEMENT_3D('',#16534,#12919,#12920);
#10490=AXIS2_PLACEMENT_3D('',#16535,#12921,#12922);
#10491=AXIS2_PLACEMENT_3D('',#16537,#12923,#12924);
#10492=AXIS2_PLACEMENT_3D('',#16538,#12925,#12926);
#10493=AXIS2_PLACEMENT_3D('',#16539,#12927,#12928);
#10494=AXIS2_PLACEMENT_3D('',#16563,#12929,#12930);
#10495=AXIS2_PLACEMENT_3D('',#16564,#12931,#12932);
#10496=AXIS2_PLACEMENT_3D('',#16566,#12933,#12934);
#10497=AXIS2_PLACEMENT_3D('',#16569,#12936,#12937);
#10498=AXIS2_PLACEMENT_3D('',#16593,#12938,#12939);
#10499=AXIS2_PLACEMENT_3D('',#16594,#12940,#12941);
#10500=AXIS2_PLACEMENT_3D('',#16595,#12942,#12943);
#10501=AXIS2_PLACEMENT_3D('',#16596,#12944,#12945);
#10502=AXIS2_PLACEMENT_3D('',#16597,#12946,#12947);
#10503=AXIS2_PLACEMENT_3D('',#16598,#12948,#12949);
#10504=AXIS2_PLACEMENT_3D('',#16599,#12950,#12951);
#12842=DIRECTION('axis',(0.,0.,1.));
#12843=DIRECTION('refdir',(1.,0.,0.));
#12844=DIRECTION('center_axis',(0.,0.,1.));
#12845=DIRECTION('ref_axis',(1.,0.,0.));
#12846=DIRECTION('center_axis',(0.,-1.,0.));
#12847=DIRECTION('ref_axis',(0.,0.,-1.));
#12848=DIRECTION('center_axis',(0.,-1.,0.));
#12849=DIRECTION('ref_axis',(0.,0.,-1.));
#12850=DIRECTION('center_axis',(0.,1.,0.));
#12851=DIRECTION('ref_axis',(1.,0.,0.));
#12852=DIRECTION('center_axis',(0.,1.,0.));
#12853=DIRECTION('ref_axis',(1.,0.,0.));
#12854=DIRECTION('center_axis',(0.,1.,0.));
#12855=DIRECTION('ref_axis',(1.,0.,0.));
#12856=DIRECTION('center_axis',(0.,1.,0.));
#12857=DIRECTION('ref_axis',(1.,0.,0.));
#12858=DIRECTION('',(0.,-1.,0.));
#12859=DIRECTION('center_axis',(0.,-1.,0.));
#12860=DIRECTION('ref_axis',(1.,0.,0.));
#12861=DIRECTION('center_axis',(0.,1.,0.));
#12862=DIRECTION('ref_axis',(1.,0.,0.));
#12863=DIRECTION('center_axis',(0.,1.,0.));
#12864=DIRECTION('ref_axis',(1.,0.,0.));
#12865=DIRECTION('center_axis',(0.,1.,0.));
#12866=DIRECTION('ref_axis',(1.,0.,0.));
#12867=DIRECTION('center_axis',(0.,1.,0.));
#12868=DIRECTION('ref_axis',(1.,0.,0.));
#12869=DIRECTION('center_axis',(0.,1.,0.));
#12870=DIRECTION('ref_axis',(1.,0.,0.));
#12871=DIRECTION('center_axis',(0.,1.,0.));
#12872=DIRECTION('ref_axis',(1.,0.,0.));
#12873=DIRECTION('center_axis',(0.,-1.,0.));
#12874=DIRECTION('ref_axis',(1.,0.,0.));
#12875=DIRECTION('center_axis',(0.,-1.,0.));
#12876=DIRECTION('ref_axis',(0.,0.,-1.));
#12877=DIRECTION('center_axis',(6.12323399573677E-17,0.,1.));
#12878=DIRECTION('ref_axis',(1.,0.,0.));
#12879=DIRECTION('center_axis',(0.,-1.,0.));
#12880=DIRECTION('ref_axis',(0.,0.,-1.));
#12881=DIRECTION('center_axis',(0.,1.,0.));
#12882=DIRECTION('ref_axis',(1.,0.,0.));
#12883=DIRECTION('center_axis',(0.,-1.,0.));
#12884=DIRECTION('ref_axis',(1.,0.,0.));
#12885=DIRECTION('center_axis',(0.,-1.,0.));
#12886=DIRECTION('ref_axis',(0.,0.,-1.));
#12887=DIRECTION('center_axis',(0.,0.,1.));
#12888=DIRECTION('ref_axis',(1.,0.,0.));
#12889=DIRECTION('center_axis',(0.,-1.,0.));
#12890=DIRECTION('ref_axis',(0.,0.,-1.));
#12891=DIRECTION('center_axis',(0.,1.,0.));
#12892=DIRECTION('ref_axis',(1.,0.,0.));
#12893=DIRECTION('center_axis',(0.,-1.,0.));
#12894=DIRECTION('ref_axis',(1.,0.,0.));
#12895=DIRECTION('center_axis',(0.,-1.,0.));
#12896=DIRECTION('ref_axis',(0.,0.,-1.));
#12897=DIRECTION('center_axis',(0.,0.,1.));
#12898=DIRECTION('ref_axis',(1.,0.,0.));
#12899=DIRECTION('center_axis',(0.,-1.,0.));
#12900=DIRECTION('ref_axis',(0.,0.,-1.));
#12901=DIRECTION('center_axis',(0.,1.,0.));
#12902=DIRECTION('ref_axis',(1.,0.,0.));
#12903=DIRECTION('center_axis',(0.,-1.,0.));
#12904=DIRECTION('ref_axis',(1.,0.,0.));
#12905=DIRECTION('center_axis',(0.,-1.,0.));
#12906=DIRECTION('ref_axis',(0.,0.,-1.));
#12907=DIRECTION('center_axis',(0.,0.,1.));
#12908=DIRECTION('ref_axis',(1.,0.,0.));
#12909=DIRECTION('center_axis',(0.,-1.,0.));
#12910=DIRECTION('ref_axis',(0.,0.,-1.));
#12911=DIRECTION('center_axis',(0.,1.,0.));
#12912=DIRECTION('ref_axis',(1.,0.,0.));
#12913=DIRECTION('center_axis',(0.,-1.,0.));
#12914=DIRECTION('ref_axis',(1.,0.,0.));
#12915=DIRECTION('center_axis',(0.,-1.,0.));
#12916=DIRECTION('ref_axis',(0.,0.,-1.));
#12917=DIRECTION('center_axis',(6.12323399573676E-17,0.,1.));
#12918=DIRECTION('ref_axis',(1.,0.,0.));
#12919=DIRECTION('center_axis',(0.,-1.,0.));
#12920=DIRECTION('ref_axis',(0.,0.,-1.));
#12921=DIRECTION('center_axis',(0.,1.,0.));
#12922=DIRECTION('ref_axis',(1.,0.,0.));
#12923=DIRECTION('center_axis',(0.,-1.,0.));
#12924=DIRECTION('ref_axis',(1.,0.,0.));
#12925=DIRECTION('center_axis',(0.,-1.,0.));
#12926=DIRECTION('ref_axis',(0.,0.,-1.));
#12927=DIRECTION('center_axis',(0.,0.,1.));
#12928=DIRECTION('ref_axis',(1.,0.,0.));
#12929=DIRECTION('center_axis',(0.,-1.,0.));
#12930=DIRECTION('ref_axis',(0.,0.,-1.));
#12931=DIRECTION('center_axis',(0.,1.,0.));
#12932=DIRECTION('ref_axis',(1.,0.,0.));
#12933=DIRECTION('center_axis',(0.,1.,0.));
#12934=DIRECTION('ref_axis',(1.,0.,0.));
#12935=DIRECTION('',(0.,1.,0.));
#12936=DIRECTION('center_axis',(0.,-1.,0.));
#12937=DIRECTION('ref_axis',(1.,0.,0.));
#12938=DIRECTION('center_axis',(0.,-1.,0.));
#12939=DIRECTION('ref_axis',(1.,0.,0.));
#12940=DIRECTION('center_axis',(0.,1.,0.));
#12941=DIRECTION('ref_axis',(1.,0.,0.));
#12942=DIRECTION('center_axis',(0.,-1.,0.));
#12943=DIRECTION('ref_axis',(0.,0.,-1.));
#12944=DIRECTION('center_axis',(0.,0.,1.));
#12945=DIRECTION('ref_axis',(1.,0.,0.));
#12946=DIRECTION('center_axis',(0.,-1.,0.));
#12947=DIRECTION('ref_axis',(0.,0.,-1.));
#12948=DIRECTION('center_axis',(0.,-1.,0.));
#12949=DIRECTION('ref_axis',(-1.,0.,0.));
#12950=DIRECTION('center_axis',(0.,1.,0.));
#12951=DIRECTION('ref_axis',(1.,0.,0.));
#16152=CARTESIAN_POINT('',(0.,0.,0.));
#16153=CARTESIAN_POINT('Origin',(0.707106781186547,0.,0.707106781186548));
#16154=CARTESIAN_POINT('',(0.504455939115715,-0.04763,0.841298510752802));
#16155=CARTESIAN_POINT('',(0.841298510752802,-0.04763,0.504455939115715));
#16156=CARTESIAN_POINT('Ctrl Pts',(0.504455939115715,-0.04763,0.841298510752802));
#16157=CARTESIAN_POINT('Ctrl Pts',(0.508899795931835,-0.0740444353928835,
0.838633903678357));
#16158=CARTESIAN_POINT('Ctrl Pts',(0.517157748491652,-0.0999305678883309,
0.833661031856294));
#16159=CARTESIAN_POINT('Ctrl Pts',(0.537715343527944,-0.142345102874864,
0.820511285096538));
#16160=CARTESIAN_POINT('Ctrl Pts',(0.548874290046456,-0.159766064500479,
0.813159949759));
#16161=CARTESIAN_POINT('Ctrl Pts',(0.573915184558107,-0.190326085855194,
0.795684265985089));
#16162=CARTESIAN_POINT('Ctrl Pts',(0.587792702767295,-0.203463743702801,
0.78555112003688));
#16163=CARTESIAN_POINT('Ctrl Pts',(0.615966552324775,-0.224161999508995,
0.763642258217233));
#16164=CARTESIAN_POINT('Ctrl Pts',(0.631684198665438,-0.232861760990032,
0.750785745543687));
#16165=CARTESIAN_POINT('Ctrl Pts',(0.663382628119203,-0.244251601209411,
0.722929908501543));
#16166=CARTESIAN_POINT('Ctrl Pts',(0.679352081686668,-0.246942143572133,
0.707917883896095));
#16167=CARTESIAN_POINT('Ctrl Pts',(0.707917883896095,-0.246942143572133,
0.679352081686668));
#16168=CARTESIAN_POINT('Ctrl Pts',(0.722929908501543,-0.244251601209411,
0.663382628119203));
#16169=CARTESIAN_POINT('Ctrl Pts',(0.750785745543687,-0.232861760990032,
0.631684198665439));
#16170=CARTESIAN_POINT('Ctrl Pts',(0.763642258217232,-0.224161999508995,
0.615966552324775));
#16171=CARTESIAN_POINT('Ctrl Pts',(0.78555112003688,-0.203463743702801,
0.587792702767295));
#16172=CARTESIAN_POINT('Ctrl Pts',(0.795684265985088,-0.190326085855194,
0.573915184558108));
#16173=CARTESIAN_POINT('Ctrl Pts',(0.813159949759,-0.15976606450048,0.548874290046456));
#16174=CARTESIAN_POINT('Ctrl Pts',(0.820511285096538,-0.142345102874864,
0.537715343527944));
#16175=CARTESIAN_POINT('Ctrl Pts',(0.833661031856294,-0.099930567888331,
0.517157748491653));
#16176=CARTESIAN_POINT('Ctrl Pts',(0.838633903678357,-0.0740444353928835,
0.508899795931835));
#16177=CARTESIAN_POINT('Ctrl Pts',(0.841298510752801,-0.0476299999999999,
0.504455939115715));
#16178=CARTESIAN_POINT('',(0.528110872004958,-0.04763,0.871530771444223));
#16179=CARTESIAN_POINT('Origin',(0.707106781186547,-0.04763,0.707106781186548));
#16180=CARTESIAN_POINT('',(0.871530771444223,-0.04763,0.528110872004959));
#16181=CARTESIAN_POINT('Ctrl Pts',(0.871530771444223,-0.0476300000000001,
0.528110872004958));
#16182=CARTESIAN_POINT('Ctrl Pts',(0.87014664509073,-0.0609922781173483,
0.530395067942936));
#16183=CARTESIAN_POINT('Ctrl Pts',(0.868149331745851,-0.0742967091364493,
0.533674141594226));
#16184=CARTESIAN_POINT('Ctrl Pts',(0.85981294420286,-0.115492077056649,
0.54708917182331));
#16185=CARTESIAN_POINT('Ctrl Pts',(0.850993704737257,-0.141695629206859,
0.560922177770136));
#16186=CARTESIAN_POINT('Ctrl Pts',(0.830754510485543,-0.181890537957859,
0.590422647829571));
#16187=CARTESIAN_POINT('Ctrl Pts',(0.816896541396381,-0.201072148666545,
0.609616703125488));
#16188=CARTESIAN_POINT('Ctrl Pts',(0.792310597819928,-0.223955109275652,
0.641117951819998));
#16189=CARTESIAN_POINT('Ctrl Pts',(0.779109323683612,-0.232742381310829,
0.657208095763053));
#16190=CARTESIAN_POINT('Ctrl Pts',(0.750552691816206,-0.244234834628584,
0.68964083160521));
#16191=CARTESIAN_POINT('Ctrl Pts',(0.735185187071673,-0.246942143572133,
0.705971972091755));
#16192=CARTESIAN_POINT('Ctrl Pts',(0.705971972091754,-0.246942143572133,
0.735185187071673));
#16193=CARTESIAN_POINT('Ctrl Pts',(0.689640831605209,-0.244234834628584,
0.750552691816206));
#16194=CARTESIAN_POINT('Ctrl Pts',(0.657208095763052,-0.232742381310829,
0.779109323683612));
#16195=CARTESIAN_POINT('Ctrl Pts',(0.641117951819998,-0.223955109275652,
0.792310597819928));
#16196=CARTESIAN_POINT('Ctrl Pts',(0.609616703125487,-0.201072148666545,
0.816896541396382));
#16197=CARTESIAN_POINT('Ctrl Pts',(0.590422647829571,-0.181890537957858,
0.830754510485544));
#16198=CARTESIAN_POINT('Ctrl Pts',(0.560922177770135,-0.141695629206858,
0.850993704737257));
#16199=CARTESIAN_POINT('Ctrl Pts',(0.547089171823309,-0.115492077056649,
0.859812944202861));
#16200=CARTESIAN_POINT('Ctrl Pts',(0.533674141594226,-0.0742967091364491,
0.868149331745852));
#16201=CARTESIAN_POINT('Ctrl Pts',(0.530395067942936,-0.0609922781173483,
0.870146645090731));
#16202=CARTESIAN_POINT('Ctrl Pts',(0.528110872004958,-0.0476300000000001,
0.871530771444223));
#16203=CARTESIAN_POINT('Origin',(0.707106781186547,-0.04763,0.707106781186548));
#16204=CARTESIAN_POINT('Origin',(0.,-0.166705,0.));
#16205=CARTESIAN_POINT('',(0.242834539687906,-0.04763,0.989696097314));
#16206=CARTESIAN_POINT('Origin',(0.,-0.04763,0.));
#16207=CARTESIAN_POINT('',(-0.242834539687907,-0.04763,0.989696097314));
#16208=CARTESIAN_POINT('Ctrl Pts',(0.242834539687906,-0.04763,0.989696097314));
#16209=CARTESIAN_POINT('Ctrl Pts',(0.24024064412003,-0.0609922781173483,
0.990332542620729));
#16210=CARTESIAN_POINT('Ctrl Pts',(0.236509675094874,-0.0742967091364492,
0.991238884025248));
#16211=CARTESIAN_POINT('Ctrl Pts',(0.221129100087819,-0.115492077056649,
0.994830026707808));
#16212=CARTESIAN_POINT('Ctrl Pts',(0.205111543747588,-0.141695629206859,
0.998375294985966));
#16213=CARTESIAN_POINT('Ctrl Pts',(0.169940289819232,-0.181890537957859,
1.00492400591205));
#16214=CARTESIAN_POINT('Ctrl Pts',(0.1465689792446,-0.201072148666545,1.00869718865384));
#16215=CARTESIAN_POINT('Ctrl Pts',(0.106909345252087,-0.223955109275652,
1.01358704779679));
#16216=CARTESIAN_POINT('Ctrl Pts',(0.0861971848975941,-0.232742381310829,
1.0156297872271));
#16217=CARTESIAN_POINT('Ctrl Pts',(0.0430711894098822,-0.244234834628584,
1.01837060663223));
#16218=CARTESIAN_POINT('Ctrl Pts',(0.0206568624125605,-0.246942143572133,
1.019052));
#16219=CARTESIAN_POINT('Ctrl Pts',(-0.0206568624125608,-0.246942143572133,
1.019052));
#16220=CARTESIAN_POINT('Ctrl Pts',(-0.0430711894098825,-0.244234834628584,
1.01837060663223));
#16221=CARTESIAN_POINT('Ctrl Pts',(-0.0861971848975943,-0.232742381310829,
1.0156297872271));
#16222=CARTESIAN_POINT('Ctrl Pts',(-0.106909345252088,-0.223955109275652,
1.01358704779679));
#16223=CARTESIAN_POINT('Ctrl Pts',(-0.1465689792446,-0.201072148666545,
1.00869718865384));
#16224=CARTESIAN_POINT('Ctrl Pts',(-0.169940289819232,-0.181890537957859,
1.00492400591205));
#16225=CARTESIAN_POINT('Ctrl Pts',(-0.205111543747588,-0.141695629206859,
0.998375294985966));
#16226=CARTESIAN_POINT('Ctrl Pts',(-0.221129100087819,-0.115492077056649,
0.994830026707808));
#16227=CARTESIAN_POINT('Ctrl Pts',(-0.236509675094875,-0.0742967091364493,
0.991238884025248));
#16228=CARTESIAN_POINT('Ctrl Pts',(-0.24024064412003,-0.0609922781173483,
0.990332542620729));
#16229=CARTESIAN_POINT('Ctrl Pts',(-0.242834539687907,-0.04763,0.989696097314));
#16230=CARTESIAN_POINT('',(-0.528110872004959,-0.04763,0.871530771444223));
#16231=CARTESIAN_POINT('Origin',(0.,-0.04763,0.));
#16232=CARTESIAN_POINT('',(-0.871530771444223,-0.04763,0.528110872004958));
#16233=CARTESIAN_POINT('Ctrl Pts',(-0.528110872004958,-0.0476300000000001,
0.871530771444223));
#16234=CARTESIAN_POINT('Ctrl Pts',(-0.530395067942936,-0.0609922781173484,
0.87014664509073));
#16235=CARTESIAN_POINT('Ctrl Pts',(-0.533674141594226,-0.0742967091364493,
0.868149331745851));
#16236=CARTESIAN_POINT('Ctrl Pts',(-0.54708917182331,-0.115492077056649,
0.85981294420286));
#16237=CARTESIAN_POINT('Ctrl Pts',(-0.560922177770136,-0.141695629206859,
0.850993704737257));
#16238=CARTESIAN_POINT('Ctrl Pts',(-0.590422647829571,-0.181890537957859,
0.830754510485543));
#16239=CARTESIAN_POINT('Ctrl Pts',(-0.609616703125488,-0.201072148666545,
0.816896541396381));
#16240=CARTESIAN_POINT('Ctrl Pts',(-0.641117951819998,-0.223955109275652,
0.792310597819928));
#16241=CARTESIAN_POINT('Ctrl Pts',(-0.657208095763053,-0.232742381310829,
0.779109323683611));
#16242=CARTESIAN_POINT('Ctrl Pts',(-0.68964083160521,-0.244234834628584,
0.750552691816205));
#16243=CARTESIAN_POINT('Ctrl Pts',(-0.705971972091755,-0.246942143572133,
0.735185187071673));
#16244=CARTESIAN_POINT('Ctrl Pts',(-0.735185187071673,-0.246942143572133,
0.705971972091754));
#16245=CARTESIAN_POINT('Ctrl Pts',(-0.750552691816206,-0.244234834628584,
0.689640831605209));
#16246=CARTESIAN_POINT('Ctrl Pts',(-0.779109323683612,-0.232742381310829,
0.657208095763052));
#16247=CARTESIAN_POINT('Ctrl Pts',(-0.792310597819928,-0.223955109275652,
0.641117951819998));
#16248=CARTESIAN_POINT('Ctrl Pts',(-0.816896541396382,-0.201072148666545,
0.609616703125487));
#16249=CARTESIAN_POINT('Ctrl Pts',(-0.830754510485544,-0.181890537957858,
0.590422647829571));
#16250=CARTESIAN_POINT('Ctrl Pts',(-0.850993704737257,-0.141695629206858,
0.560922177770135));
#16251=CARTESIAN_POINT('Ctrl Pts',(-0.859812944202861,-0.115492077056649,
0.547089171823309));
#16252=CARTESIAN_POINT('Ctrl Pts',(-0.868149331745852,-0.0742967091364491,
0.533674141594226));
#16253=CARTESIAN_POINT('Ctrl Pts',(-0.870146645090731,-0.0609922781173483,
0.530395067942936));
#16254=CARTESIAN_POINT('Ctrl Pts',(-0.871530771444223,-0.04763,0.528110872004958));
#16255=CARTESIAN_POINT('',(-0.989696097314,-0.04763,0.242834539687906));
#16256=CARTESIAN_POINT('Origin',(0.,-0.04763,0.));
#16257=CARTESIAN_POINT('',(-1.019052,-0.246942143572133,1.248489836334E-16));
#16258=CARTESIAN_POINT('Ctrl Pts',(-0.989696097314,-0.04763,0.242834539687906));
#16259=CARTESIAN_POINT('Ctrl Pts',(-0.990332542620729,-0.0609922781173483,
0.24024064412003));
#16260=CARTESIAN_POINT('Ctrl Pts',(-0.991238884025248,-0.0742967091364492,
0.236509675094874));
#16261=CARTESIAN_POINT('Ctrl Pts',(-0.994830026707808,-0.115492077056649,
0.221129100087819));
#16262=CARTESIAN_POINT('Ctrl Pts',(-0.998375294985966,-0.141695629206859,
0.205111543747588));
#16263=CARTESIAN_POINT('Ctrl Pts',(-1.00492400591205,-0.181890537957859,
0.169940289819232));
#16264=CARTESIAN_POINT('Ctrl Pts',(-1.00869718865384,-0.201072148666545,
0.1465689792446));
#16265=CARTESIAN_POINT('Ctrl Pts',(-1.01358704779679,-0.223955109275652,
0.106909345252088));
#16266=CARTESIAN_POINT('Ctrl Pts',(-1.0156297872271,-0.232742381310829,
0.0861971848975944));
#16267=CARTESIAN_POINT('Ctrl Pts',(-1.01837060663223,-0.244234834628584,
0.0430711894098825));
#16268=CARTESIAN_POINT('Ctrl Pts',(-1.019052,-0.246942143572133,0.0206568624125608));
#16269=CARTESIAN_POINT('Ctrl Pts',(-1.019052,-0.246942143572133,1.2490009027033E-16));
#16270=CARTESIAN_POINT('',(-1.019052,-0.28578,1.24797876996471E-16));
#16271=CARTESIAN_POINT('',(-1.019052,-0.166705,1.24797876996471E-16));
#16272=CARTESIAN_POINT('Origin',(0.,-0.28578,0.));
#16273=CARTESIAN_POINT('',(-0.989696097314,-0.04763,-0.242834539687906));
#16274=CARTESIAN_POINT('Ctrl Pts',(-1.019052,-0.246942143572133,1.2490009027033E-16));
#16275=CARTESIAN_POINT('Ctrl Pts',(-1.019052,-0.246942143572133,-0.0206568624125605));
#16276=CARTESIAN_POINT('Ctrl Pts',(-1.01837060663223,-0.244234834628584,
-0.0430711894098822));
#16277=CARTESIAN_POINT('Ctrl Pts',(-1.0156297872271,-0.232742381310829,
-0.0861971848975941));
#16278=CARTESIAN_POINT('Ctrl Pts',(-1.01358704779679,-0.223955109275652,
-0.106909345252087));
#16279=CARTESIAN_POINT('Ctrl Pts',(-1.00869718865384,-0.201072148666546,
-0.1465689792446));
#16280=CARTESIAN_POINT('Ctrl Pts',(-1.00492400591205,-0.181890537957859,
-0.169940289819232));
#16281=CARTESIAN_POINT('Ctrl Pts',(-0.998375294985966,-0.141695629206859,
-0.205111543747588));
#16282=CARTESIAN_POINT('Ctrl Pts',(-0.994830026707808,-0.11549207705665,
-0.221129100087819));
#16283=CARTESIAN_POINT('Ctrl Pts',(-0.991238884025248,-0.0742967091364495,
-0.236509675094874));
#16284=CARTESIAN_POINT('Ctrl Pts',(-0.990332542620729,-0.0609922781173484,
-0.24024064412003));
#16285=CARTESIAN_POINT('Ctrl Pts',(-0.989696097314,-0.0476300000000001,
-0.242834539687907));
#16286=CARTESIAN_POINT('',(-0.871530771444223,-0.04763,-0.528110872004958));
#16287=CARTESIAN_POINT('Origin',(0.,-0.04763,0.));
#16288=CARTESIAN_POINT('',(-0.528110872004958,-0.04763,-0.871530771444223));
#16289=CARTESIAN_POINT('Ctrl Pts',(-0.871530771444223,-0.0476300000000001,
-0.528110872004958));
#16290=CARTESIAN_POINT('Ctrl Pts',(-0.87014664509073,-0.0609922781173484,
-0.530395067942936));
#16291=CARTESIAN_POINT('Ctrl Pts',(-0.868149331745851,-0.0742967091364494,
-0.533674141594226));
#16292=CARTESIAN_POINT('Ctrl Pts',(-0.85981294420286,-0.115492077056649,
-0.54708917182331));
#16293=CARTESIAN_POINT('Ctrl Pts',(-0.850993704737257,-0.141695629206859,
-0.560922177770136));
#16294=CARTESIAN_POINT('Ctrl Pts',(-0.830754510485543,-0.181890537957859,
-0.590422647829571));
#16295=CARTESIAN_POINT('Ctrl Pts',(-0.816896541396381,-0.201072148666546,
-0.609616703125488));
#16296=CARTESIAN_POINT('Ctrl Pts',(-0.792310597819928,-0.223955109275652,
-0.641117951819999));
#16297=CARTESIAN_POINT('Ctrl Pts',(-0.779109323683611,-0.232742381310829,
-0.657208095763053));
#16298=CARTESIAN_POINT('Ctrl Pts',(-0.750552691816205,-0.244234834628584,
-0.68964083160521));
#16299=CARTESIAN_POINT('Ctrl Pts',(-0.735185187071673,-0.246942143572133,
-0.705971972091755));
#16300=CARTESIAN_POINT('Ctrl Pts',(-0.705971972091754,-0.246942143572133,
-0.735185187071673));
#16301=CARTESIAN_POINT('Ctrl Pts',(-0.68964083160521,-0.244234834628584,
-0.750552691816206));
#16302=CARTESIAN_POINT('Ctrl Pts',(-0.657208095763052,-0.232742381310829,
-0.779109323683612));
#16303=CARTESIAN_POINT('Ctrl Pts',(-0.641117951819998,-0.223955109275652,
-0.792310597819928));
#16304=CARTESIAN_POINT('Ctrl Pts',(-0.609616703125488,-0.201072148666545,
-0.816896541396381));
#16305=CARTESIAN_POINT('Ctrl Pts',(-0.590422647829571,-0.181890537957859,
-0.830754510485543));
#16306=CARTESIAN_POINT('Ctrl Pts',(-0.560922177770136,-0.141695629206859,
-0.850993704737257));
#16307=CARTESIAN_POINT('Ctrl Pts',(-0.54708917182331,-0.115492077056649,
-0.85981294420286));
#16308=CARTESIAN_POINT('Ctrl Pts',(-0.533674141594226,-0.0742967091364494,
-0.868149331745852));
#16309=CARTESIAN_POINT('Ctrl Pts',(-0.530395067942936,-0.0609922781173484,
-0.870146645090731));
#16310=CARTESIAN_POINT('Ctrl Pts',(-0.528110872004958,-0.0476300000000001,
-0.871530771444223));
#16311=CARTESIAN_POINT('',(-0.242834539687906,-0.04763,-0.989696097314));
#16312=CARTESIAN_POINT('Origin',(0.,-0.04763,0.));
#16313=CARTESIAN_POINT('',(0.242834539687906,-0.04763,-0.989696097314));
#16314=CARTESIAN_POINT('Ctrl Pts',(-0.242834539687907,-0.04763,-0.989696097314));
#16315=CARTESIAN_POINT('Ctrl Pts',(-0.24024064412003,-0.0609922781173483,
-0.990332542620729));
#16316=CARTESIAN_POINT('Ctrl Pts',(-0.236509675094874,-0.0742967091364493,
-0.991238884025248));
#16317=CARTESIAN_POINT('Ctrl Pts',(-0.221129100087819,-0.115492077056649,
-0.994830026707808));
#16318=CARTESIAN_POINT('Ctrl Pts',(-0.205111543747588,-0.141695629206859,
-0.998375294985966));
#16319=CARTESIAN_POINT('Ctrl Pts',(-0.169940289819232,-0.181890537957859,
-1.00492400591205));
#16320=CARTESIAN_POINT('Ctrl Pts',(-0.1465689792446,-0.201072148666545,
-1.00869718865384));
#16321=CARTESIAN_POINT('Ctrl Pts',(-0.106909345252087,-0.223955109275652,
-1.01358704779679));
#16322=CARTESIAN_POINT('Ctrl Pts',(-0.0861971848975942,-0.232742381310829,
-1.0156297872271));
#16323=CARTESIAN_POINT('Ctrl Pts',(-0.0430711894098823,-0.244234834628584,
-1.01837060663223));
#16324=CARTESIAN_POINT('Ctrl Pts',(-0.0206568624125606,-0.246942143572133,
-1.019052));
#16325=CARTESIAN_POINT('Ctrl Pts',(0.0206568624125607,-0.246942143572133,
-1.019052));
#16326=CARTESIAN_POINT('Ctrl Pts',(0.0430711894098824,-0.244234834628584,
-1.01837060663223));
#16327=CARTESIAN_POINT('Ctrl Pts',(0.0861971848975943,-0.232742381310829,
-1.0156297872271));
#16328=CARTESIAN_POINT('Ctrl Pts',(0.106909345252088,-0.223955109275652,
-1.01358704779679));
#16329=CARTESIAN_POINT('Ctrl Pts',(0.1465689792446,-0.201072148666545,-1.00869718865384));
#16330=CARTESIAN_POINT('Ctrl Pts',(0.169940289819232,-0.181890537957859,
-1.00492400591205));
#16331=CARTESIAN_POINT('Ctrl Pts',(0.205111543747588,-0.141695629206859,
-0.998375294985966));
#16332=CARTESIAN_POINT('Ctrl Pts',(0.221129100087819,-0.115492077056649,
-0.994830026707808));
#16333=CARTESIAN_POINT('Ctrl Pts',(0.236509675094874,-0.0742967091364493,
-0.991238884025248));
#16334=CARTESIAN_POINT('Ctrl Pts',(0.24024064412003,-0.0609922781173484,
-0.990332542620729));
#16335=CARTESIAN_POINT('Ctrl Pts',(0.242834539687907,-0.04763,-0.989696097314));
#16336=CARTESIAN_POINT('',(0.528110872004958,-0.04763,-0.871530771444223));
#16337=CARTESIAN_POINT('Origin',(0.,-0.04763,0.));
#16338=CARTESIAN_POINT('',(0.871530771444223,-0.04763,-0.528110872004958));
#16339=CARTESIAN_POINT('Ctrl Pts',(0.528110872004958,-0.0476300000000001,
-0.871530771444223));
#16340=CARTESIAN_POINT('Ctrl Pts',(0.530395067942936,-0.0609922781173484,
-0.870146645090731));
#16341=CARTESIAN_POINT('Ctrl Pts',(0.533674141594226,-0.0742967091364493,
-0.868149331745851));
#16342=CARTESIAN_POINT('Ctrl Pts',(0.54708917182331,-0.115492077056649,
-0.85981294420286));
#16343=CARTESIAN_POINT('Ctrl Pts',(0.560922177770136,-0.141695629206859,
-0.850993704737257));
#16344=CARTESIAN_POINT('Ctrl Pts',(0.590422647829571,-0.181890537957859,
-0.830754510485543));
#16345=CARTESIAN_POINT('Ctrl Pts',(0.609616703125488,-0.201072148666545,
-0.816896541396381));
#16346=CARTESIAN_POINT('Ctrl Pts',(0.641117951819998,-0.223955109275652,
-0.792310597819928));
#16347=CARTESIAN_POINT('Ctrl Pts',(0.657208095763053,-0.232742381310829,
-0.779109323683612));
#16348=CARTESIAN_POINT('Ctrl Pts',(0.68964083160521,-0.244234834628584,
-0.750552691816206));
#16349=CARTESIAN_POINT('Ctrl Pts',(0.705971972091755,-0.246942143572133,
-0.735185187071673));
#16350=CARTESIAN_POINT('Ctrl Pts',(0.735185187071673,-0.246942143572133,
-0.705971972091754));
#16351=CARTESIAN_POINT('Ctrl Pts',(0.750552691816206,-0.244234834628584,
-0.68964083160521));
#16352=CARTESIAN_POINT('Ctrl Pts',(0.779109323683612,-0.232742381310829,
-0.657208095763053));
#16353=CARTESIAN_POINT('Ctrl Pts',(0.792310597819928,-0.223955109275652,
-0.641117951819998));
#16354=CARTESIAN_POINT('Ctrl Pts',(0.816896541396381,-0.201072148666545,
-0.609616703125488));
#16355=CARTESIAN_POINT('Ctrl Pts',(0.830754510485543,-0.181890537957859,
-0.590422647829571));
#16356=CARTESIAN_POINT('Ctrl Pts',(0.850993704737257,-0.141695629206859,
-0.560922177770136));
#16357=CARTESIAN_POINT('Ctrl Pts',(0.85981294420286,-0.115492077056649,
-0.54708917182331));
#16358=CARTESIAN_POINT('Ctrl Pts',(0.868149331745851,-0.0742967091364493,
-0.533674141594226));
#16359=CARTESIAN_POINT('Ctrl Pts',(0.870146645090731,-0.0609922781173484,
-0.530395067942936));
#16360=CARTESIAN_POINT('Ctrl Pts',(0.871530771444223,-0.0476300000000001,
-0.528110872004958));
#16361=CARTESIAN_POINT('',(0.989696097314,-0.04763,-0.242834539687906));
#16362=CARTESIAN_POINT('Origin',(0.,-0.04763,0.));
#16363=CARTESIAN_POINT('',(0.989696097314,-0.04763,0.242834539687906));
#16364=CARTESIAN_POINT('Ctrl Pts',(0.989696097314,-0.04763,-0.242834539687907));
#16365=CARTESIAN_POINT('Ctrl Pts',(0.990332542620729,-0.0609922781173483,
-0.24024064412003));
#16366=CARTESIAN_POINT('Ctrl Pts',(0.991238884025248,-0.0742967091364493,
-0.236509675094874));
#16367=CARTESIAN_POINT('Ctrl Pts',(0.994830026707808,-0.115492077056649,
-0.221129100087819));
#16368=CARTESIAN_POINT('Ctrl Pts',(0.998375294985966,-0.141695629206859,
-0.205111543747588));
#16369=CARTESIAN_POINT('Ctrl Pts',(1.00492400591205,-0.181890537957859,
-0.169940289819232));
#16370=CARTESIAN_POINT('Ctrl Pts',(1.00869718865384,-0.201072148666545,
-0.1465689792446));
#16371=CARTESIAN_POINT('Ctrl Pts',(1.01358704779679,-0.223955109275652,
-0.106909345252087));
#16372=CARTESIAN_POINT('Ctrl Pts',(1.0156297872271,-0.232742381310829,-0.0861971848975942));
#16373=CARTESIAN_POINT('Ctrl Pts',(1.01837060663223,-0.244234834628584,
-0.0430711894098823));
#16374=CARTESIAN_POINT('Ctrl Pts',(1.019052,-0.246942143572133,-0.0206568624125607));
#16375=CARTESIAN_POINT('Ctrl Pts',(1.019052,-0.246942143572133,0.0206568624125607));
#16376=CARTESIAN_POINT('Ctrl Pts',(1.01837060663223,-0.244234834628584,
0.0430711894098823));
#16377=CARTESIAN_POINT('Ctrl Pts',(1.0156297872271,-0.232742381310829,0.0861971848975942));
#16378=CARTESIAN_POINT('Ctrl Pts',(1.01358704779679,-0.223955109275652,
0.106909345252087));
#16379=CARTESIAN_POINT('Ctrl Pts',(1.00869718865384,-0.201072148666545,
0.1465689792446));
#16380=CARTESIAN_POINT('Ctrl Pts',(1.00492400591205,-0.181890537957859,
0.169940289819232));
#16381=CARTESIAN_POINT('Ctrl Pts',(0.998375294985966,-0.141695629206859,
0.205111543747588));
#16382=CARTESIAN_POINT('Ctrl Pts',(0.994830026707808,-0.115492077056649,
0.221129100087819));
#16383=CARTESIAN_POINT('Ctrl Pts',(0.991238884025248,-0.0742967091364492,
0.236509675094874));
#16384=CARTESIAN_POINT('Ctrl Pts',(0.990332542620729,-0.0609922781173483,
0.24024064412003));
#16385=CARTESIAN_POINT('Ctrl Pts',(0.989696097314,-0.04763,0.242834539687907));
#16386=CARTESIAN_POINT('Origin',(0.,-0.04763,0.));
#16387=CARTESIAN_POINT('Origin',(0.,-0.04763,0.));
#16388=CARTESIAN_POINT('',(0.238183666596899,-0.04763,0.951592097314));
#16389=CARTESIAN_POINT('Origin',(0.,-0.04763,0.));
#16390=CARTESIAN_POINT('Origin',(-1.94289029309402E-16,-0.04763,1.));
#16391=CARTESIAN_POINT('Origin',(-1.94289029309402E-16,0.,1.));
#16392=CARTESIAN_POINT('',(-0.2381836665969,-0.04763,0.951592097314));
#16393=CARTESIAN_POINT('Ctrl Pts',(-0.238183666596899,-0.0476299999999999,
0.951592097314));
#16394=CARTESIAN_POINT('Ctrl Pts',(-0.233157223576062,-0.0740444353928835,
0.952850216871763));
#16395=CARTESIAN_POINT('Ctrl Pts',(-0.223801617934946,-0.0999305678883309,
0.955173119738174));
#16396=CARTESIAN_POINT('Ctrl Pts',(-0.199966927975188,-0.142345102874864,
0.960411259488514));
#16397=CARTESIAN_POINT('Ctrl Pts',(-0.1868781821531,-0.159766064500479,
0.963103647174702));
#16398=CARTESIAN_POINT('Ctrl Pts',(-0.15681442133453,-0.190326085855194,
0.968453058988463));
#16399=CARTESIAN_POINT('Ctrl Pts',(-0.139836317888043,-0.203463743702801,
0.971100730005489));
#16400=CARTESIAN_POINT('Ctrl Pts',(-0.104422493053067,-0.224161999508995,
0.975530745318961));
#16401=CARTESIAN_POINT('Ctrl Pts',(-0.0842175114474176,-0.232861760990032,
0.977553872336861));
#16402=CARTESIAN_POINT('Ctrl Pts',(-0.0421062857595701,-0.244251601209411,
0.980270995488453));
#16403=CARTESIAN_POINT('Ctrl Pts',(-0.0201990724523197,-0.246942143572133,
0.980948));
#16404=CARTESIAN_POINT('Ctrl Pts',(0.020199072452319,-0.246942143572133,
0.980948));
#16405=CARTESIAN_POINT('Ctrl Pts',(0.0421062857595694,-0.244251601209411,
0.980270995488454));
#16406=CARTESIAN_POINT('Ctrl Pts',(0.0842175114474169,-0.232861760990032,
0.977553872336861));
#16407=CARTESIAN_POINT('Ctrl Pts',(0.104422493053067,-0.224161999508995,
0.975530745318961));
#16408=CARTESIAN_POINT('Ctrl Pts',(0.139836317888042,-0.203463743702801,
0.971100730005489));
#16409=CARTESIAN_POINT('Ctrl Pts',(0.15681442133453,-0.190326085855194,
0.968453058988463));
#16410=CARTESIAN_POINT('Ctrl Pts',(0.1868781821531,-0.15976606450048,0.963103647174702));
#16411=CARTESIAN_POINT('Ctrl Pts',(0.199966927975188,-0.142345102874864,
0.960411259488514));
#16412=CARTESIAN_POINT('Ctrl Pts',(0.223801617934945,-0.0999305678883309,
0.955173119738174));
#16413=CARTESIAN_POINT('Ctrl Pts',(0.233157223576061,-0.0740444353928835,
0.952850216871763));
#16414=CARTESIAN_POINT('Ctrl Pts',(0.238183666596899,-0.0476299999999999,
0.951592097314));
#16415=CARTESIAN_POINT('Origin',(-1.94289029309402E-16,-0.04763,1.));
#16416=CARTESIAN_POINT('Origin',(0.,-0.04763,0.));
#16417=CARTESIAN_POINT('',(-0.504455939115715,-0.04763,0.841298510752802));
#16418=CARTESIAN_POINT('Origin',(0.,-0.04763,0.));
#16419=CARTESIAN_POINT('Origin',(-0.707106781186548,-0.04763,0.707106781186547));
#16420=CARTESIAN_POINT('Origin',(-0.707106781186548,0.,0.707106781186547));
#16421=CARTESIAN_POINT('',(-0.841298510752802,-0.04763,0.504455939115715));
#16422=CARTESIAN_POINT('Ctrl Pts',(-0.841298510752802,-0.04763,0.504455939115715));
#16423=CARTESIAN_POINT('Ctrl Pts',(-0.838633903678357,-0.0740444353928835,
0.508899795931835));
#16424=CARTESIAN_POINT('Ctrl Pts',(-0.833661031856294,-0.0999305678883309,
0.517157748491652));
#16425=CARTESIAN_POINT('Ctrl Pts',(-0.820511285096538,-0.142345102874864,
0.537715343527944));
#16426=CARTESIAN_POINT('Ctrl Pts',(-0.813159949759,-0.159766064500479,0.548874290046456));
#16427=CARTESIAN_POINT('Ctrl Pts',(-0.795684265985089,-0.190326085855194,
0.573915184558107));
#16428=CARTESIAN_POINT('Ctrl Pts',(-0.78555112003688,-0.203463743702801,
0.587792702767295));
#16429=CARTESIAN_POINT('Ctrl Pts',(-0.763642258217233,-0.224161999508995,
0.615966552324775));
#16430=CARTESIAN_POINT('Ctrl Pts',(-0.750785745543687,-0.232861760990032,
0.631684198665438));
#16431=CARTESIAN_POINT('Ctrl Pts',(-0.722929908501543,-0.244251601209411,
0.663382628119203));
#16432=CARTESIAN_POINT('Ctrl Pts',(-0.707917883896095,-0.246942143572133,
0.679352081686668));
#16433=CARTESIAN_POINT('Ctrl Pts',(-0.679352081686668,-0.246942143572133,
0.707917883896095));
#16434=CARTESIAN_POINT('Ctrl Pts',(-0.663382628119203,-0.244251601209411,
0.722929908501544));
#16435=CARTESIAN_POINT('Ctrl Pts',(-0.631684198665438,-0.232861760990031,
0.750785745543687));
#16436=CARTESIAN_POINT('Ctrl Pts',(-0.615966552324775,-0.224161999508995,
0.763642258217233));
#16437=CARTESIAN_POINT('Ctrl Pts',(-0.587792702767295,-0.203463743702801,
0.78555112003688));
#16438=CARTESIAN_POINT('Ctrl Pts',(-0.573915184558107,-0.190326085855194,
0.795684265985088));
#16439=CARTESIAN_POINT('Ctrl Pts',(-0.548874290046456,-0.159766064500479,
0.813159949759));
#16440=CARTESIAN_POINT('Ctrl Pts',(-0.537715343527944,-0.142345102874864,
0.820511285096538));
#16441=CARTESIAN_POINT('Ctrl Pts',(-0.517157748491652,-0.0999305678883309,
0.833661031856294));
#16442=CARTESIAN_POINT('Ctrl Pts',(-0.508899795931835,-0.0740444353928835,
0.838633903678357));
#16443=CARTESIAN_POINT('Ctrl Pts',(-0.504455939115716,-0.04763,0.841298510752801));
#16444=CARTESIAN_POINT('Origin',(-0.707106781186548,-0.04763,0.707106781186547));
#16445=CARTESIAN_POINT('Origin',(0.,-0.04763,0.));
#16446=CARTESIAN_POINT('',(-0.951592097314,-0.04763,0.238183666596899));
#16447=CARTESIAN_POINT('Origin',(0.,-0.04763,0.));
#16448=CARTESIAN_POINT('Origin',(-1.,-0.04763,-1.11022302462516E-16));
#16449=CARTESIAN_POINT('Origin',(-1.,0.,-1.11022302462516E-16));
#16450=CARTESIAN_POINT('',(-0.951592097314,-0.04763,-0.2381836665969));
#16451=CARTESIAN_POINT('',(-0.980948,-0.246942143572133,1.08514323328844E-18));
#16452=CARTESIAN_POINT('Ctrl Pts',(-0.951592097314,-0.04763,-0.238183666596899));
#16453=CARTESIAN_POINT('Ctrl Pts',(-0.952850216871763,-0.0740444353928835,
-0.233157223576062));
#16454=CARTESIAN_POINT('Ctrl Pts',(-0.955173119738174,-0.0999305678883309,
-0.223801617934946));
#16455=CARTESIAN_POINT('Ctrl Pts',(-0.960411259488514,-0.142345102874864,
-0.199966927975188));
#16456=CARTESIAN_POINT('Ctrl Pts',(-0.963103647174702,-0.159766064500479,
-0.1868781821531));
#16457=CARTESIAN_POINT('Ctrl Pts',(-0.968453058988463,-0.190326085855194,
-0.15681442133453));
#16458=CARTESIAN_POINT('Ctrl Pts',(-0.971100730005489,-0.203463743702801,
-0.139836317888043));
#16459=CARTESIAN_POINT('Ctrl Pts',(-0.975530745318961,-0.224161999508995,
-0.104422493053067));
#16460=CARTESIAN_POINT('Ctrl Pts',(-0.977553872336861,-0.232861760990032,
-0.0842175114474175));
#16461=CARTESIAN_POINT('Ctrl Pts',(-0.980270995488453,-0.244251601209411,
-0.0421062857595699));
#16462=CARTESIAN_POINT('Ctrl Pts',(-0.980948,-0.246942143572133,-0.0201990724523195));
#16463=CARTESIAN_POINT('Ctrl Pts',(-0.980948,-0.246942143572133,-1.17961196366423E-16));
#16464=CARTESIAN_POINT('Origin',(-1.,-0.04763,-1.11022302462516E-16));
#16465=CARTESIAN_POINT('Ctrl Pts',(-0.980948,-0.246942143572133,-1.17961196366423E-16));
#16466=CARTESIAN_POINT('Ctrl Pts',(-0.980948,-0.246942143572133,0.0201990724523192));
#16467=CARTESIAN_POINT('Ctrl Pts',(-0.980270995488453,-0.244251601209411,
0.0421062857595695));
#16468=CARTESIAN_POINT('Ctrl Pts',(-0.977553872336861,-0.232861760990032,
0.0842175114474169));
#16469=CARTESIAN_POINT('Ctrl Pts',(-0.975530745318961,-0.224161999508995,
0.104422493053066));
#16470=CARTESIAN_POINT('Ctrl Pts',(-0.971100730005489,-0.203463743702801,
0.139836317888042));
#16471=CARTESIAN_POINT('Ctrl Pts',(-0.968453058988463,-0.190326085855194,
0.15681442133453));
#16472=CARTESIAN_POINT('Ctrl Pts',(-0.963103647174702,-0.15976606450048,
0.1868781821531));
#16473=CARTESIAN_POINT('Ctrl Pts',(-0.960411259488514,-0.142345102874864,
0.199966927975188));
#16474=CARTESIAN_POINT('Ctrl Pts',(-0.955173119738174,-0.099930567888331,
0.223801617934945));
#16475=CARTESIAN_POINT('Ctrl Pts',(-0.952850216871763,-0.0740444353928835,
0.233157223576061));
#16476=CARTESIAN_POINT('Ctrl Pts',(-0.951592097314,-0.04763,0.238183666596899));
#16477=CARTESIAN_POINT('Origin',(0.,-0.04763,0.));
#16478=CARTESIAN_POINT('',(-0.841298510752802,-0.04763,-0.504455939115715));
#16479=CARTESIAN_POINT('Origin',(0.,-0.04763,0.));
#16480=CARTESIAN_POINT('Origin',(-0.707106781186547,-0.04763,-0.707106781186548));
#16481=CARTESIAN_POINT('Origin',(-0.707106781186547,0.,-0.707106781186548));
#16482=CARTESIAN_POINT('',(-0.504455939115715,-0.04763,-0.841298510752802));
#16483=CARTESIAN_POINT('Ctrl Pts',(-0.504455939115715,-0.04763,-0.841298510752802));
#16484=CARTESIAN_POINT('Ctrl Pts',(-0.508899795931835,-0.0740444353928835,
-0.838633903678357));
#16485=CARTESIAN_POINT('Ctrl Pts',(-0.517157748491652,-0.0999305678883309,
-0.833661031856294));
#16486=CARTESIAN_POINT('Ctrl Pts',(-0.537715343527944,-0.142345102874864,
-0.820511285096538));
#16487=CARTESIAN_POINT('Ctrl Pts',(-0.548874290046456,-0.159766064500479,
-0.813159949759));
#16488=CARTESIAN_POINT('Ctrl Pts',(-0.573915184558107,-0.190326085855194,
-0.795684265985089));
#16489=CARTESIAN_POINT('Ctrl Pts',(-0.587792702767295,-0.203463743702801,
-0.78555112003688));
#16490=CARTESIAN_POINT('Ctrl Pts',(-0.615966552324775,-0.224161999508995,
-0.763642258217233));
#16491=CARTESIAN_POINT('Ctrl Pts',(-0.631684198665438,-0.232861760990032,
-0.750785745543687));
#16492=CARTESIAN_POINT('Ctrl Pts',(-0.663382628119203,-0.244251601209411,
-0.722929908501543));
#16493=CARTESIAN_POINT('Ctrl Pts',(-0.679352081686668,-0.246942143572133,
-0.707917883896095));
#16494=CARTESIAN_POINT('Ctrl Pts',(-0.707917883896095,-0.246942143572133,
-0.679352081686668));
#16495=CARTESIAN_POINT('Ctrl Pts',(-0.722929908501543,-0.244251601209411,
-0.663382628119203));
#16496=CARTESIAN_POINT('Ctrl Pts',(-0.750785745543687,-0.232861760990032,
-0.631684198665439));
#16497=CARTESIAN_POINT('Ctrl Pts',(-0.763642258217232,-0.224161999508995,
-0.615966552324775));
#16498=CARTESIAN_POINT('Ctrl Pts',(-0.78555112003688,-0.203463743702801,
-0.587792702767295));
#16499=CARTESIAN_POINT('Ctrl Pts',(-0.795684265985088,-0.190326085855194,
-0.573915184558107));
#16500=CARTESIAN_POINT('Ctrl Pts',(-0.813159949759,-0.15976606450048,-0.548874290046456));
#16501=CARTESIAN_POINT('Ctrl Pts',(-0.820511285096538,-0.142345102874864,
-0.537715343527944));
#16502=CARTESIAN_POINT('Ctrl Pts',(-0.833661031856294,-0.0999305678883311,
-0.517157748491652));
#16503=CARTESIAN_POINT('Ctrl Pts',(-0.838633903678357,-0.0740444353928836,
-0.508899795931835));
#16504=CARTESIAN_POINT('Ctrl Pts',(-0.841298510752801,-0.04763,-0.504455939115715));
#16505=CARTESIAN_POINT('Origin',(-0.707106781186547,-0.04763,-0.707106781186548));
#16506=CARTESIAN_POINT('Origin',(0.,-0.04763,0.));
#16507=CARTESIAN_POINT('',(-0.238183666596899,-0.04763,-0.951592097314));
#16508=CARTESIAN_POINT('Origin',(0.,-0.04763,0.));
#16509=CARTESIAN_POINT('Origin',(5.55111512312578E-17,-0.04763,-1.));
#16510=CARTESIAN_POINT('Origin',(5.55111512312578E-17,0.,-1.));
#16511=CARTESIAN_POINT('',(0.238183666596899,-0.04763,-0.951592097314));
#16512=CARTESIAN_POINT('Ctrl Pts',(0.238183666596899,-0.04763,-0.951592097314));
#16513=CARTESIAN_POINT('Ctrl Pts',(0.233157223576062,-0.0740444353928835,
-0.952850216871763));
#16514=CARTESIAN_POINT('Ctrl Pts',(0.223801617934946,-0.099930567888331,
-0.955173119738174));
#16515=CARTESIAN_POINT('Ctrl Pts',(0.199966927975188,-0.142345102874864,
-0.960411259488514));
#16516=CARTESIAN_POINT('Ctrl Pts',(0.1868781821531,-0.15976606450048,-0.963103647174702));
#16517=CARTESIAN_POINT('Ctrl Pts',(0.15681442133453,-0.190326085855194,
-0.968453058988463));
#16518=CARTESIAN_POINT('Ctrl Pts',(0.139836317888042,-0.203463743702801,
-0.971100730005489));
#16519=CARTESIAN_POINT('Ctrl Pts',(0.104422493053067,-0.224161999508995,
-0.975530745318961));
#16520=CARTESIAN_POINT('Ctrl Pts',(0.0842175114474173,-0.232861760990032,
-0.977553872336861));
#16521=CARTESIAN_POINT('Ctrl Pts',(0.0421062857595698,-0.244251601209411,
-0.980270995488453));
#16522=CARTESIAN_POINT('Ctrl Pts',(0.0201990724523194,-0.246942143572133,
-0.980948));
#16523=CARTESIAN_POINT('Ctrl Pts',(-0.0201990724523193,-0.246942143572133,
-0.980948));
#16524=CARTESIAN_POINT('Ctrl Pts',(-0.0421062857595697,-0.244251601209411,
-0.980270995488453));
#16525=CARTESIAN_POINT('Ctrl Pts',(-0.0842175114474171,-0.232861760990032,
-0.977553872336861));
#16526=CARTESIAN_POINT('Ctrl Pts',(-0.104422493053067,-0.224161999508995,
-0.975530745318961));
#16527=CARTESIAN_POINT('Ctrl Pts',(-0.139836317888042,-0.203463743702801,
-0.971100730005489));
#16528=CARTESIAN_POINT('Ctrl Pts',(-0.15681442133453,-0.190326085855194,
-0.968453058988463));
#16529=CARTESIAN_POINT('Ctrl Pts',(-0.1868781821531,-0.15976606450048,-0.963103647174702));
#16530=CARTESIAN_POINT('Ctrl Pts',(-0.199966927975188,-0.142345102874864,
-0.960411259488514));
#16531=CARTESIAN_POINT('Ctrl Pts',(-0.223801617934945,-0.099930567888331,
-0.955173119738174));
#16532=CARTESIAN_POINT('Ctrl Pts',(-0.233157223576062,-0.0740444353928835,
-0.952850216871763));
#16533=CARTESIAN_POINT('Ctrl Pts',(-0.238183666596899,-0.0476299999999999,
-0.951592097314));
#16534=CARTESIAN_POINT('Origin',(5.55111512312578E-17,-0.04763,-1.));
#16535=CARTESIAN_POINT('Origin',(0.,-0.04763,0.));
#16536=CARTESIAN_POINT('',(0.504455939115715,-0.04763,-0.841298510752802));
#16537=CARTESIAN_POINT('Origin',(0.,-0.04763,0.));
#16538=CARTESIAN_POINT('Origin',(0.707106781186548,-0.04763,-0.707106781186547));
#16539=CARTESIAN_POINT('Origin',(0.707106781186548,0.,-0.707106781186547));
#16540=CARTESIAN_POINT('',(0.841298510752802,-0.04763,-0.504455939115715));
#16541=CARTESIAN_POINT('Ctrl Pts',(0.841298510752802,-0.04763,-0.504455939115715));
#16542=CARTESIAN_POINT('Ctrl Pts',(0.838633903678357,-0.0740444353928835,
-0.508899795931835));
#16543=CARTESIAN_POINT('Ctrl Pts',(0.833661031856294,-0.0999305678883309,
-0.517157748491652));
#16544=CARTESIAN_POINT('Ctrl Pts',(0.820511285096538,-0.142345102874864,
-0.537715343527944));
#16545=CARTESIAN_POINT('Ctrl Pts',(0.813159949759,-0.159766064500479,-0.548874290046456));
#16546=CARTESIAN_POINT('Ctrl Pts',(0.795684265985088,-0.190326085855194,
-0.573915184558107));
#16547=CARTESIAN_POINT('Ctrl Pts',(0.78555112003688,-0.203463743702801,
-0.587792702767295));
#16548=CARTESIAN_POINT('Ctrl Pts',(0.763642258217233,-0.224161999508995,
-0.615966552324775));
#16549=CARTESIAN_POINT('Ctrl Pts',(0.750785745543687,-0.232861760990032,
-0.631684198665438));
#16550=CARTESIAN_POINT('Ctrl Pts',(0.722929908501543,-0.244251601209411,
-0.663382628119203));
#16551=CARTESIAN_POINT('Ctrl Pts',(0.707917883896095,-0.246942143572133,
-0.679352081686668));
#16552=CARTESIAN_POINT('Ctrl Pts',(0.679352081686668,-0.246942143572133,
-0.707917883896095));
#16553=CARTESIAN_POINT('Ctrl Pts',(0.663382628119203,-0.244251601209411,
-0.722929908501543));
#16554=CARTESIAN_POINT('Ctrl Pts',(0.631684198665438,-0.232861760990032,
-0.750785745543687));
#16555=CARTESIAN_POINT('Ctrl Pts',(0.615966552324775,-0.224161999508995,
-0.763642258217232));
#16556=CARTESIAN_POINT('Ctrl Pts',(0.587792702767295,-0.203463743702801,
-0.78555112003688));
#16557=CARTESIAN_POINT('Ctrl Pts',(0.573915184558107,-0.190326085855194,
-0.795684265985088));
#16558=CARTESIAN_POINT('Ctrl Pts',(0.548874290046456,-0.159766064500479,
-0.813159949759));
#16559=CARTESIAN_POINT('Ctrl Pts',(0.537715343527944,-0.142345102874864,
-0.820511285096538));
#16560=CARTESIAN_POINT('Ctrl Pts',(0.517157748491652,-0.099930567888331,
-0.833661031856294));
#16561=CARTESIAN_POINT('Ctrl Pts',(0.508899795931835,-0.0740444353928835,
-0.838633903678357));
#16562=CARTESIAN_POINT('Ctrl Pts',(0.504455939115715,-0.04763,-0.841298510752801));
#16563=CARTESIAN_POINT('Origin',(0.707106781186548,-0.04763,-0.707106781186547));
#16564=CARTESIAN_POINT('Origin',(0.,-0.166705,0.));
#16565=CARTESIAN_POINT('',(-0.980948,-0.28578,1.20131482833E-16));
#16566=CARTESIAN_POINT('Origin',(0.,-0.28578,0.));
#16567=CARTESIAN_POINT('',(-0.980948,-0.166705,1.20131482833E-16));
#16568=CARTESIAN_POINT('',(0.951592097314,-0.04763,0.238183666596899));
#16569=CARTESIAN_POINT('Origin',(0.,-0.04763,0.));
#16570=CARTESIAN_POINT('',(0.951592097314,-0.04763,-0.238183666596899));
#16571=CARTESIAN_POINT('Ctrl Pts',(0.951592097314,-0.04763,0.238183666596899));
#16572=CARTESIAN_POINT('Ctrl Pts',(0.952850216871763,-0.0740444353928835,
0.233157223576062));
#16573=CARTESIAN_POINT('Ctrl Pts',(0.955173119738174,-0.099930567888331,
0.223801617934945));
#16574=CARTESIAN_POINT('Ctrl Pts',(0.960411259488514,-0.142345102874864,
0.199966927975188));
#16575=CARTESIAN_POINT('Ctrl Pts',(0.963103647174702,-0.15976606450048,
0.1868781821531));
#16576=CARTESIAN_POINT('Ctrl Pts',(0.968453058988463,-0.190326085855194,
0.15681442133453));
#16577=CARTESIAN_POINT('Ctrl Pts',(0.971100730005489,-0.203463743702801,
0.139836317888042));
#16578=CARTESIAN_POINT('Ctrl Pts',(0.975530745318961,-0.224161999508995,
0.104422493053067));
#16579=CARTESIAN_POINT('Ctrl Pts',(0.977553872336861,-0.232861760990032,
0.0842175114474172));
#16580=CARTESIAN_POINT('Ctrl Pts',(0.980270995488453,-0.244251601209411,
0.0421062857595697));
#16581=CARTESIAN_POINT('Ctrl Pts',(0.980948,-0.246942143572133,0.0201990724523194));
#16582=CARTESIAN_POINT('Ctrl Pts',(0.980948,-0.246942143572133,-0.0201990724523194));
#16583=CARTESIAN_POINT('Ctrl Pts',(0.980270995488453,-0.244251601209411,
-0.0421062857595697));
#16584=CARTESIAN_POINT('Ctrl Pts',(0.977553872336861,-0.232861760990032,
-0.0842175114474172));
#16585=CARTESIAN_POINT('Ctrl Pts',(0.975530745318961,-0.224161999508995,
-0.104422493053067));
#16586=CARTESIAN_POINT('Ctrl Pts',(0.971100730005489,-0.203463743702801,
-0.139836317888042));
#16587=CARTESIAN_POINT('Ctrl Pts',(0.968453058988463,-0.190326085855194,
-0.15681442133453));
#16588=CARTESIAN_POINT('Ctrl Pts',(0.963103647174702,-0.15976606450048,
-0.1868781821531));
#16589=CARTESIAN_POINT('Ctrl Pts',(0.960411259488514,-0.142345102874864,
-0.199966927975188));
#16590=CARTESIAN_POINT('Ctrl Pts',(0.955173119738174,-0.099930567888331,
-0.223801617934945));
#16591=CARTESIAN_POINT('Ctrl Pts',(0.952850216871763,-0.0740444353928835,
-0.233157223576062));
#16592=CARTESIAN_POINT('Ctrl Pts',(0.951592097314,-0.0476299999999999,-0.238183666596899));
#16593=CARTESIAN_POINT('Origin',(0.,-0.04763,0.));
#16594=CARTESIAN_POINT('Origin',(0.,-0.04763,0.));
#16595=CARTESIAN_POINT('Origin',(1.,-0.04763,0.));
#16596=CARTESIAN_POINT('Origin',(1.,0.,0.));
#16597=CARTESIAN_POINT('Origin',(1.,-0.04763,0.));
#16598=CARTESIAN_POINT('Origin',(0.,-0.28578,0.));
#16599=CARTESIAN_POINT('Origin',(0.,-0.04763,0.));
#17247=UNCERTAINTY_MEASURE_WITH_UNIT(LENGTH_MEASURE(0.001),#17323,
'DISTANCE_ACCURACY_VALUE',
'Maximum model space distance between geometric entities at asserted c
onnectivities');
#17261=UNCERTAINTY_MEASURE_WITH_UNIT(LENGTH_MEASURE(0.001),#17323,
'DISTANCE_ACCURACY_VALUE',
'Maximum model space distance between geometric entities at asserted c
onnectivities');
#17308=(
GEOMETRIC_REPRESENTATION_CONTEXT(3)
GLOBAL_UNCERTAINTY_ASSIGNED_CONTEXT((#17247))
GLOBAL_UNIT_ASSIGNED_CONTEXT((#17323,#17325,#17326))
REPRESENTATION_CONTEXT('','3D')
);
#17322=(
GEOMETRIC_REPRESENTATION_CONTEXT(3)
GLOBAL_UNCERTAINTY_ASSIGNED_CONTEXT((#17261))
GLOBAL_UNIT_ASSIGNED_CONTEXT((#17323,#17325,#17326))
REPRESENTATION_CONTEXT('','3D')
);
#17323=(
LENGTH_UNIT()
NAMED_UNIT(*)
SI_UNIT(.CENTI.,.METRE.)
);
#17325=(
NAMED_UNIT(*)
PLANE_ANGLE_UNIT()
SI_UNIT($,.RADIAN.)
);
#17326=(
NAMED_UNIT(*)
SI_UNIT($,.STERADIAN.)
SOLID_ANGLE_UNIT()
);
#17373=SHAPE_DEFINITION_REPRESENTATION(#17435,#17604);
#17435=PRODUCT_DEFINITION_SHAPE('',$,#17665);
#17604=SHAPE_REPRESENTATION('',(#10451),#17308);
#17618=PRODUCT_DEFINITION_CONTEXT('part definition',#17800,'design');
#17665=PRODUCT_DEFINITION('Cage','Cage',#17725,#17618);
#17725=PRODUCT_DEFINITION_FORMATION('',$,#17848);
#17800=APPLICATION_CONTEXT(
'Core Data for Automotive Mechanical Design Process');
#17801=PRODUCT_CONTEXT('part definition',#17800,'mechanical');
#17848=PRODUCT('Cage','Cage','Cage',(#17801));
#17925=COLOUR_RGB('Grey',0.48,0.52,0.57);
#17926=FILL_AREA_STYLE_COLOUR('',#17925);
#17927=FILL_AREA_STYLE('',(#17926));
#17928=SURFACE_STYLE_FILL_AREA(#17927);
#17929=SURFACE_SIDE_STYLE('',(#17928));
#17930=SURFACE_STYLE_USAGE(.BOTH.,#17929);
#17931=PRESENTATION_STYLE_ASSIGNMENT((#17930));
ENDSEC;
END-ISO-10303-21;
